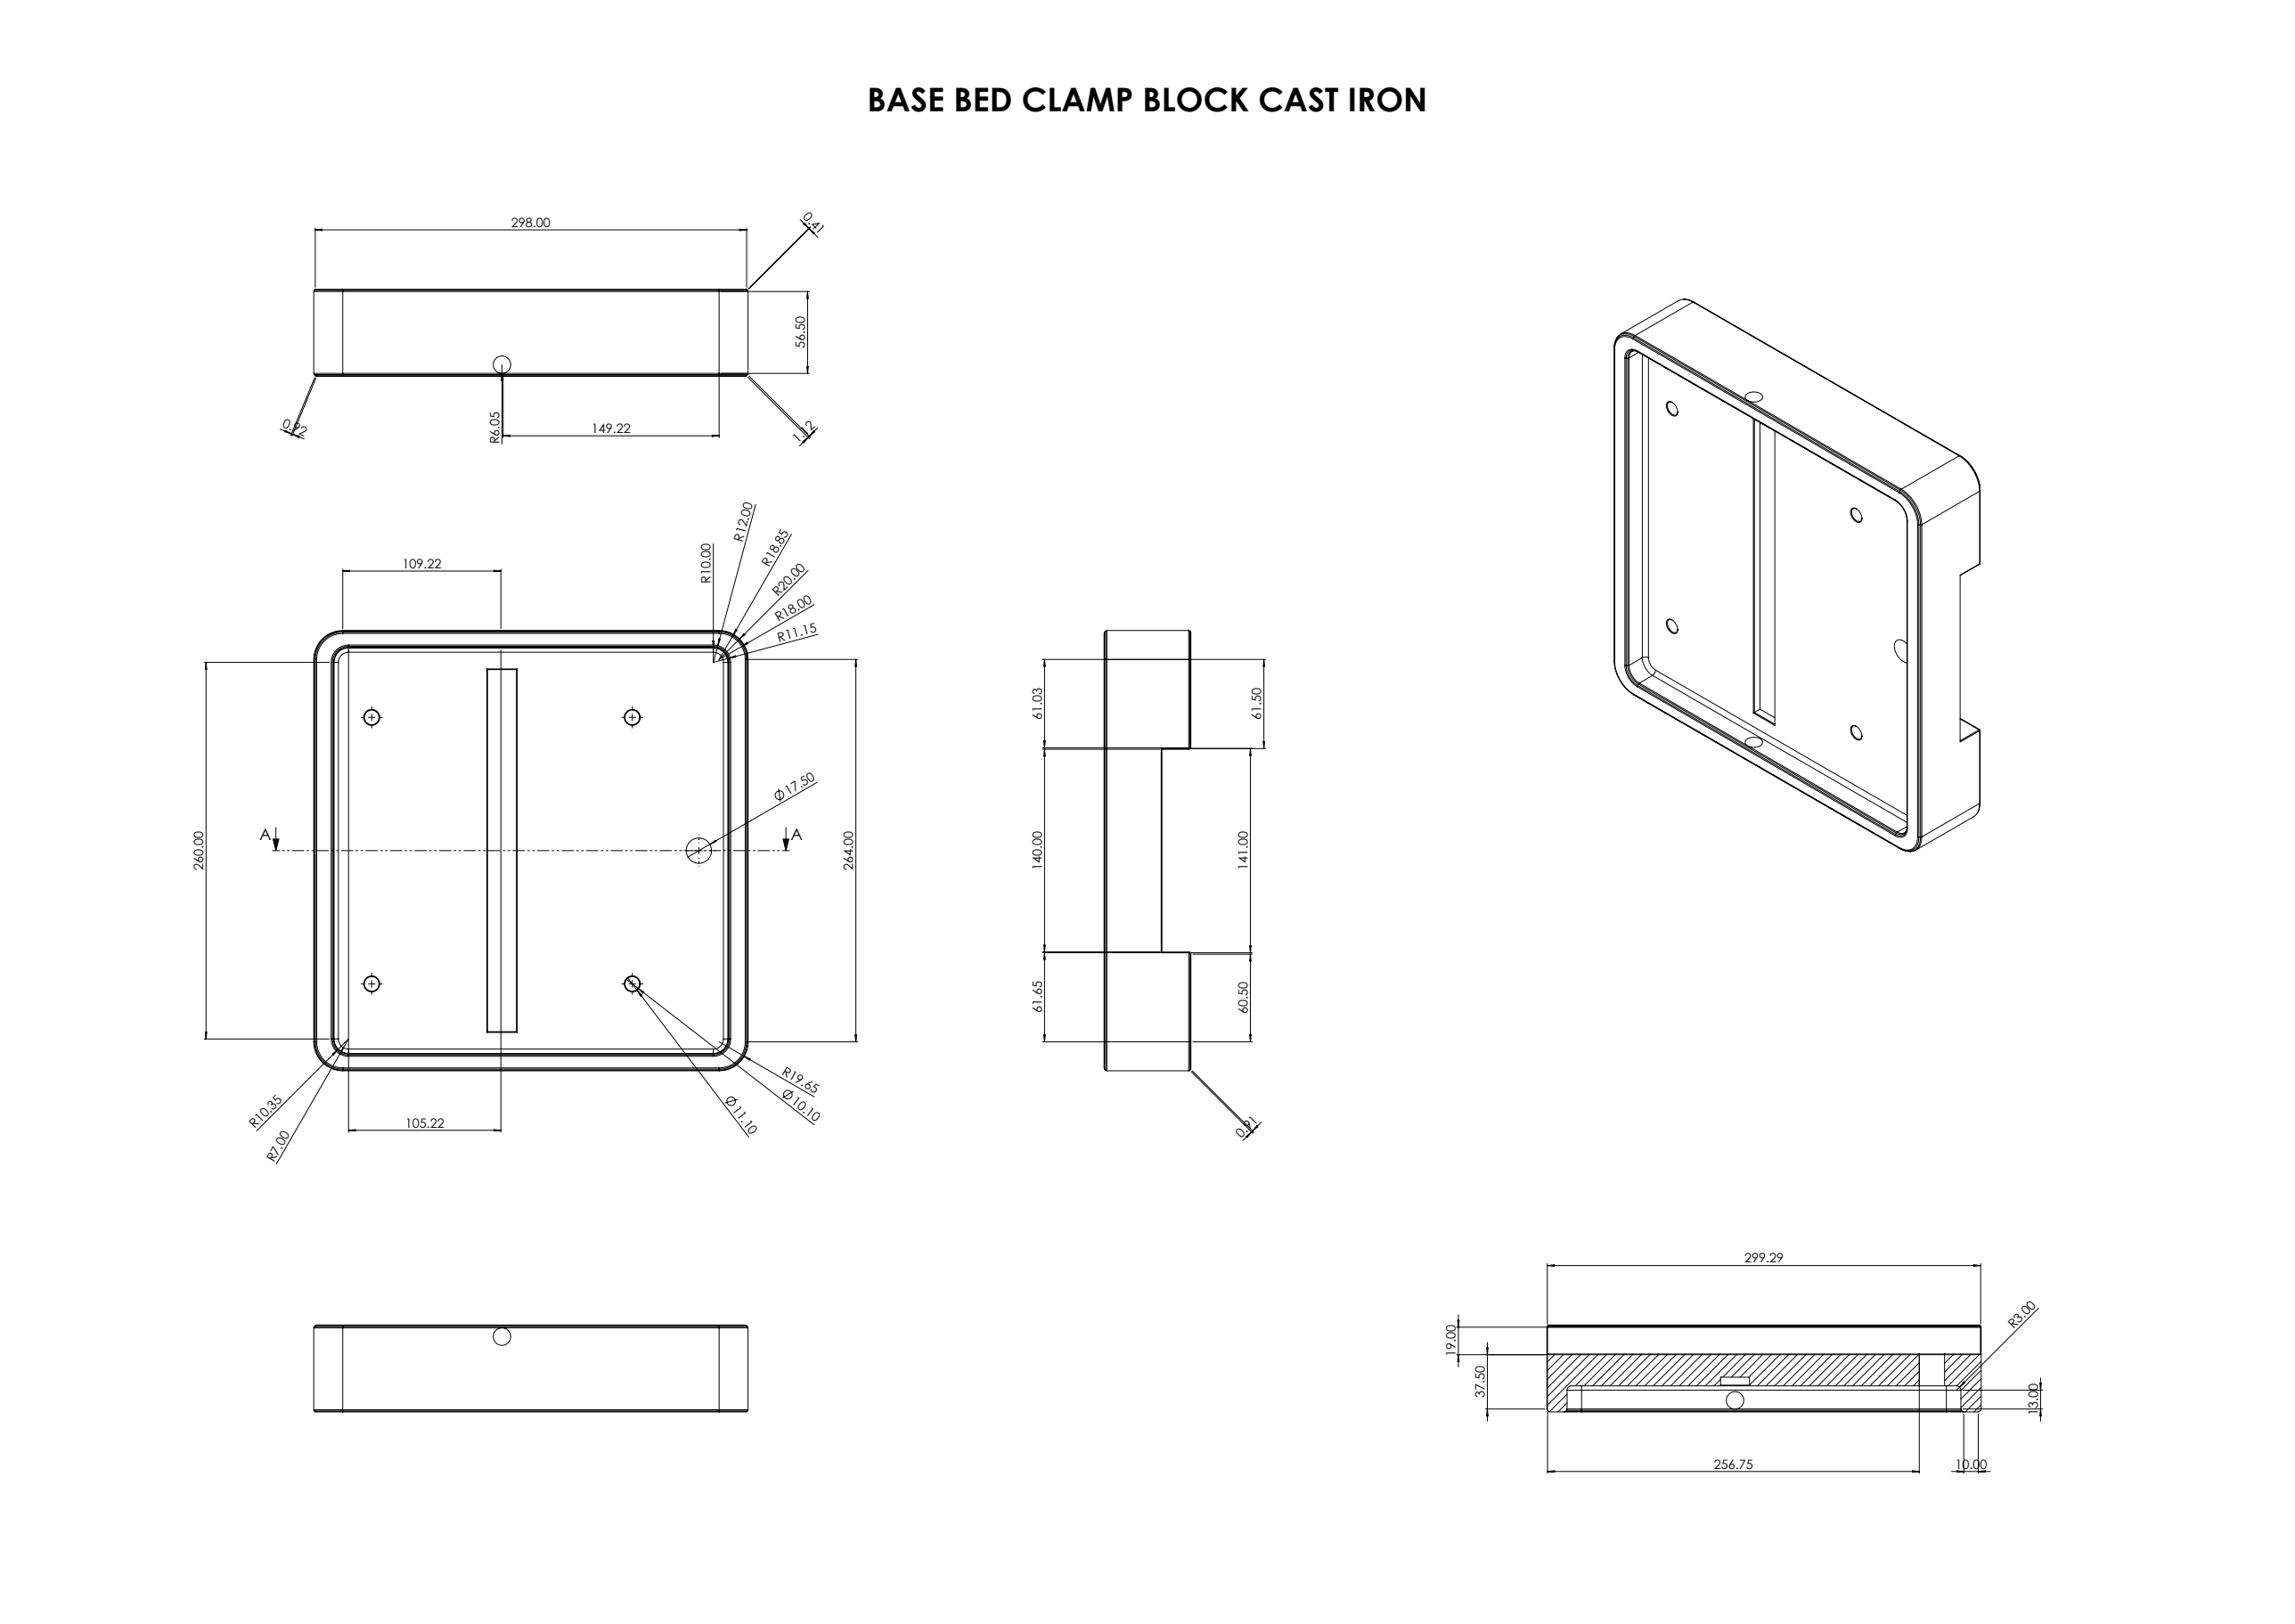
ISO-10303-21;
HEADER;
/* Generated by software containing ST-Developer
 * from STEP Tools, Inc. (www.steptools.com) 
 */

FILE_DESCRIPTION(
/* description */ (''),
/* implementation_level */ '2;1');

FILE_NAME(
/* name */ '01_Base_Bed_Clamp_Block_Cast_Iron.step',
/* time_stamp */ '2026-10-26T03:50:32-07:00',
/* author */ (''),
/* organization */ (''),
/* preprocessor_version */ 'ST-DEVELOPER v20.2',
/* originating_system */ 'Autodesk Translation Framework v15.15.0.0',
/* authorisation */ '');

FILE_SCHEMA (('AUTOMOTIVE_DESIGN { 1 0 10303 214 3 1 1 }'));
ENDSEC;

DATA;
#10=MECHANICAL_DESIGN_GEOMETRIC_PRESENTATION_REPRESENTATION('',(#1039),#76660);
#999=SHAPE_REPRESENTATION_RELATIONSHIP('SRR','None',#76736,#1019);
#1019=ADVANCED_BREP_SHAPE_REPRESENTATION('',(#1059),#76640);
#1039=STYLED_ITEM('',(#76885),#1059);
#1059=MANIFOLD_SOLID_BREP('Base',#26664);
#1079=TOROIDAL_SURFACE('',#27101,0.7,0.3);
#1080=TOROIDAL_SURFACE('',#27107,0.700000000000007,0.3);
#1081=TOROIDAL_SURFACE('',#27111,0.700000000000002,0.3);
#1082=TOROIDAL_SURFACE('',#27115,0.699999999999998,0.3);
#1089=ELLIPSE('',#26967,0.654847281176891,0.605);
#1090=ELLIPSE('',#26976,0.654847281176891,0.605);
#1091=ELLIPSE('',#26995,0.654847281176891,0.605);
#1092=ELLIPSE('',#27030,0.654847281176891,0.605);
#1103=CYLINDRICAL_SURFACE('',#26946,0.505000000000003);
#1104=CYLINDRICAL_SURFACE('',#26950,0.505000000000003);
#1105=CYLINDRICAL_SURFACE('',#26954,0.504999999999999);
#1106=CYLINDRICAL_SURFACE('',#26958,0.504999999999999);
#1107=CYLINDRICAL_SURFACE('',#26985,1.);
#1108=CYLINDRICAL_SURFACE('',#26988,1.00000000000001);
#1109=CYLINDRICAL_SURFACE('',#26993,0.605);
#1110=CYLINDRICAL_SURFACE('',#27043,2.);
#1111=CYLINDRICAL_SURFACE('',#27046,2.);
#1112=CYLINDRICAL_SURFACE('',#27105,0.3);
#1113=CYLINDRICAL_SURFACE('',#27109,0.3);
#1114=CYLINDRICAL_SURFACE('',#27113,0.3);
#1115=CYLINDRICAL_SURFACE('',#27118,0.3);
#1116=CYLINDRICAL_SURFACE('',#27119,0.999999999999998);
#1117=CYLINDRICAL_SURFACE('',#27121,1.);
#1118=CYLINDRICAL_SURFACE('',#27130,2.);
#1119=CYLINDRICAL_SURFACE('',#27131,0.605);
#1120=CYLINDRICAL_SURFACE('',#27132,0.875);
#1121=CYLINDRICAL_SURFACE('',#27140,2.);
#1553=FACE_BOUND('',#4089,.T.);
#1554=FACE_BOUND('',#4092,.T.);
#1555=FACE_BOUND('',#4093,.T.);
#1556=FACE_BOUND('',#4094,.T.);
#1557=FACE_BOUND('',#4095,.T.);
#1558=FACE_BOUND('',#4096,.T.);
#1559=FACE_BOUND('',#4097,.T.);
#1560=FACE_BOUND('',#4194,.T.);
#1656=PLANE('',#26910);
#1657=PLANE('',#26914);
#1658=PLANE('',#26918);
#1659=PLANE('',#26922);
#1660=PLANE('',#26923);
#1661=PLANE('',#26926);
#1662=PLANE('',#26929);
#1663=PLANE('',#26937);
#1664=PLANE('',#26960);
#1665=PLANE('',#26961);
#1666=PLANE('',#26962);
#1667=PLANE('',#26963);
#1668=PLANE('',#26964);
#1669=PLANE('',#26965);
#1670=PLANE('',#26966);
#1671=PLANE('',#26971);
#1672=PLANE('',#26975);
#1673=PLANE('',#26979);
#1674=PLANE('',#26982);
#1675=PLANE('',#26987);
#1676=PLANE('',#26990);
#1677=PLANE('',#26997);
#1678=PLANE('',#26998);
#1679=PLANE('',#26999);
#1680=PLANE('',#27000);
#1681=PLANE('',#27001);
#1682=PLANE('',#27002);
#1683=PLANE('',#27003);
#1684=PLANE('',#27004);
#1685=PLANE('',#27005);
#1686=PLANE('',#27006);
#1687=PLANE('',#27009);
#1688=PLANE('',#27012);
#1689=PLANE('',#27015);
#1690=PLANE('',#27018);
#1691=PLANE('',#27019);
#1692=PLANE('',#27022);
#1693=PLANE('',#27025);
#1694=PLANE('',#27029);
#1695=PLANE('',#27034);
#1696=PLANE('',#27037);
#1697=PLANE('',#27040);
#1698=PLANE('',#27045);
#1699=PLANE('',#27048);
#1700=PLANE('',#27052);
#1701=PLANE('',#27055);
#1702=PLANE('',#27058);
#1703=PLANE('',#27061);
#1704=PLANE('',#27062);
#1705=PLANE('',#27063);
#1706=PLANE('',#27067);
#1707=PLANE('',#27071);
#1708=PLANE('',#27072);
#1709=PLANE('',#27073);
#1710=PLANE('',#27074);
#1711=PLANE('',#27075);
#1712=PLANE('',#27076);
#1713=PLANE('',#27077);
#1714=PLANE('',#27080);
#1715=PLANE('',#27084);
#1716=PLANE('',#27085);
#1717=PLANE('',#27086);
#1718=PLANE('',#27087);
#1719=PLANE('',#27088);
#1720=PLANE('',#27090);
#1721=PLANE('',#27091);
#1722=PLANE('',#27093);
#1723=PLANE('',#27094);
#1724=PLANE('',#27096);
#1725=PLANE('',#27097);
#1726=PLANE('',#27098);
#1727=PLANE('',#27099);
#1728=PLANE('',#27100);
#1729=PLANE('',#27120);
#1730=PLANE('',#27123);
#1731=PLANE('',#27125);
#1732=PLANE('',#27127);
#1733=PLANE('',#27129);
#1734=PLANE('',#27137);
#1735=PLANE('',#27138);
#1736=PLANE('',#27139);
#2524=FACE_OUTER_BOUND('',#4076,.T.);
#2525=FACE_OUTER_BOUND('',#4077,.T.);
#2526=FACE_OUTER_BOUND('',#4078,.T.);
#2527=FACE_OUTER_BOUND('',#4079,.T.);
#2528=FACE_OUTER_BOUND('',#4080,.T.);
#2529=FACE_OUTER_BOUND('',#4081,.T.);
#2530=FACE_OUTER_BOUND('',#4082,.T.);
#2531=FACE_OUTER_BOUND('',#4083,.T.);
#2532=FACE_OUTER_BOUND('',#4084,.T.);
#2533=FACE_OUTER_BOUND('',#4085,.T.);
#2534=FACE_OUTER_BOUND('',#4086,.T.);
#2535=FACE_OUTER_BOUND('',#4087,.T.);
#2536=FACE_OUTER_BOUND('',#4088,.T.);
#2537=FACE_OUTER_BOUND('',#4090,.T.);
#2538=FACE_OUTER_BOUND('',#4091,.T.);
#2539=FACE_OUTER_BOUND('',#4098,.T.);
#2540=FACE_OUTER_BOUND('',#4099,.T.);
#2541=FACE_OUTER_BOUND('',#4100,.T.);
#2542=FACE_OUTER_BOUND('',#4101,.T.);
#2543=FACE_OUTER_BOUND('',#4102,.T.);
#2544=FACE_OUTER_BOUND('',#4103,.T.);
#2545=FACE_OUTER_BOUND('',#4104,.T.);
#2546=FACE_OUTER_BOUND('',#4105,.T.);
#2547=FACE_OUTER_BOUND('',#4106,.T.);
#2548=FACE_OUTER_BOUND('',#4107,.T.);
#2549=FACE_OUTER_BOUND('',#4108,.T.);
#2550=FACE_OUTER_BOUND('',#4109,.T.);
#2551=FACE_OUTER_BOUND('',#4110,.T.);
#2552=FACE_OUTER_BOUND('',#4111,.T.);
#2553=FACE_OUTER_BOUND('',#4112,.T.);
#2554=FACE_OUTER_BOUND('',#4113,.T.);
#2555=FACE_OUTER_BOUND('',#4114,.T.);
#2556=FACE_OUTER_BOUND('',#4115,.T.);
#2557=FACE_OUTER_BOUND('',#4116,.T.);
#2558=FACE_OUTER_BOUND('',#4117,.T.);
#2559=FACE_OUTER_BOUND('',#4118,.T.);
#2560=FACE_OUTER_BOUND('',#4119,.T.);
#2561=FACE_OUTER_BOUND('',#4120,.T.);
#2562=FACE_OUTER_BOUND('',#4121,.T.);
#2563=FACE_OUTER_BOUND('',#4122,.T.);
#2564=FACE_OUTER_BOUND('',#4123,.T.);
#2565=FACE_OUTER_BOUND('',#4124,.T.);
#2566=FACE_OUTER_BOUND('',#4125,.T.);
#2567=FACE_OUTER_BOUND('',#4126,.T.);
#2568=FACE_OUTER_BOUND('',#4127,.T.);
#2569=FACE_OUTER_BOUND('',#4128,.T.);
#2570=FACE_OUTER_BOUND('',#4129,.T.);
#2571=FACE_OUTER_BOUND('',#4130,.T.);
#2572=FACE_OUTER_BOUND('',#4131,.T.);
#2573=FACE_OUTER_BOUND('',#4132,.T.);
#2574=FACE_OUTER_BOUND('',#4133,.T.);
#2575=FACE_OUTER_BOUND('',#4134,.T.);
#2576=FACE_OUTER_BOUND('',#4135,.T.);
#2577=FACE_OUTER_BOUND('',#4136,.T.);
#2578=FACE_OUTER_BOUND('',#4137,.T.);
#2579=FACE_OUTER_BOUND('',#4138,.T.);
#2580=FACE_OUTER_BOUND('',#4139,.T.);
#2581=FACE_OUTER_BOUND('',#4140,.T.);
#2582=FACE_OUTER_BOUND('',#4141,.T.);
#2583=FACE_OUTER_BOUND('',#4142,.T.);
#2584=FACE_OUTER_BOUND('',#4143,.T.);
#2585=FACE_OUTER_BOUND('',#4144,.T.);
#2586=FACE_OUTER_BOUND('',#4145,.T.);
#2587=FACE_OUTER_BOUND('',#4146,.T.);
#2588=FACE_OUTER_BOUND('',#4147,.T.);
#2589=FACE_OUTER_BOUND('',#4148,.T.);
#2590=FACE_OUTER_BOUND('',#4149,.T.);
#2591=FACE_OUTER_BOUND('',#4150,.T.);
#2592=FACE_OUTER_BOUND('',#4151,.T.);
#2593=FACE_OUTER_BOUND('',#4152,.T.);
#2594=FACE_OUTER_BOUND('',#4153,.T.);
#2595=FACE_OUTER_BOUND('',#4154,.T.);
#2596=FACE_OUTER_BOUND('',#4155,.T.);
#2597=FACE_OUTER_BOUND('',#4156,.T.);
#2598=FACE_OUTER_BOUND('',#4157,.T.);
#2599=FACE_OUTER_BOUND('',#4158,.T.);
#2600=FACE_OUTER_BOUND('',#4159,.T.);
#2601=FACE_OUTER_BOUND('',#4160,.T.);
#2602=FACE_OUTER_BOUND('',#4161,.T.);
#2603=FACE_OUTER_BOUND('',#4162,.T.);
#2604=FACE_OUTER_BOUND('',#4163,.T.);
#2605=FACE_OUTER_BOUND('',#4164,.T.);
#2606=FACE_OUTER_BOUND('',#4165,.T.);
#2607=FACE_OUTER_BOUND('',#4166,.T.);
#2608=FACE_OUTER_BOUND('',#4167,.T.);
#2609=FACE_OUTER_BOUND('',#4168,.T.);
#2610=FACE_OUTER_BOUND('',#4169,.T.);
#2611=FACE_OUTER_BOUND('',#4170,.T.);
#2612=FACE_OUTER_BOUND('',#4171,.T.);
#2613=FACE_OUTER_BOUND('',#4172,.T.);
#2614=FACE_OUTER_BOUND('',#4173,.T.);
#2615=FACE_OUTER_BOUND('',#4174,.T.);
#2616=FACE_OUTER_BOUND('',#4175,.T.);
#2617=FACE_OUTER_BOUND('',#4176,.T.);
#2618=FACE_OUTER_BOUND('',#4177,.T.);
#2619=FACE_OUTER_BOUND('',#4178,.T.);
#2620=FACE_OUTER_BOUND('',#4179,.T.);
#2621=FACE_OUTER_BOUND('',#4180,.T.);
#2622=FACE_OUTER_BOUND('',#4181,.T.);
#2623=FACE_OUTER_BOUND('',#4182,.T.);
#2624=FACE_OUTER_BOUND('',#4183,.T.);
#2625=FACE_OUTER_BOUND('',#4184,.T.);
#2626=FACE_OUTER_BOUND('',#4185,.T.);
#2627=FACE_OUTER_BOUND('',#4186,.T.);
#2628=FACE_OUTER_BOUND('',#4187,.T.);
#2629=FACE_OUTER_BOUND('',#4188,.T.);
#2630=FACE_OUTER_BOUND('',#4189,.T.);
#2631=FACE_OUTER_BOUND('',#4190,.T.);
#2632=FACE_OUTER_BOUND('',#4191,.T.);
#2633=FACE_OUTER_BOUND('',#4192,.T.);
#2634=FACE_OUTER_BOUND('',#4193,.T.);
#2635=FACE_OUTER_BOUND('',#4195,.T.);
#2636=FACE_OUTER_BOUND('',#4196,.T.);
#2637=FACE_OUTER_BOUND('',#4197,.T.);
#2638=FACE_OUTER_BOUND('',#4198,.T.);
#2639=FACE_OUTER_BOUND('',#4199,.T.);
#2640=FACE_OUTER_BOUND('',#4200,.T.);
#2641=FACE_OUTER_BOUND('',#4201,.T.);
#2642=FACE_OUTER_BOUND('',#4202,.T.);
#2643=FACE_OUTER_BOUND('',#4203,.T.);
#2644=FACE_OUTER_BOUND('',#4204,.T.);
#2645=FACE_OUTER_BOUND('',#4205,.T.);
#2646=FACE_OUTER_BOUND('',#4206,.T.);
#2647=FACE_OUTER_BOUND('',#4207,.T.);
#2648=FACE_OUTER_BOUND('',#4208,.T.);
#2649=FACE_OUTER_BOUND('',#4209,.T.);
#2650=FACE_OUTER_BOUND('',#4210,.T.);
#2651=FACE_OUTER_BOUND('',#4211,.T.);
#2652=FACE_OUTER_BOUND('',#4212,.T.);
#2653=FACE_OUTER_BOUND('',#4213,.T.);
#2654=FACE_OUTER_BOUND('',#4214,.T.);
#2655=FACE_OUTER_BOUND('',#4215,.T.);
#2656=FACE_OUTER_BOUND('',#4216,.T.);
#2657=FACE_OUTER_BOUND('',#4217,.T.);
#2658=FACE_OUTER_BOUND('',#4218,.T.);
#2659=FACE_OUTER_BOUND('',#4219,.T.);
#2660=FACE_OUTER_BOUND('',#4220,.T.);
#2661=FACE_OUTER_BOUND('',#4221,.T.);
#2662=FACE_OUTER_BOUND('',#4222,.T.);
#2663=FACE_OUTER_BOUND('',#4223,.T.);
#2664=FACE_OUTER_BOUND('',#4224,.T.);
#2665=FACE_OUTER_BOUND('',#4225,.T.);
#2666=FACE_OUTER_BOUND('',#4226,.T.);
#2667=FACE_OUTER_BOUND('',#4227,.T.);
#2668=FACE_OUTER_BOUND('',#4228,.T.);
#2669=FACE_OUTER_BOUND('',#4229,.T.);
#4076=EDGE_LOOP('',(#17185,#17186,#17187,#17188));
#4077=EDGE_LOOP('',(#17189,#17190,#17191,#17192));
#4078=EDGE_LOOP('',(#17193,#17194,#17195,#17196));
#4079=EDGE_LOOP('',(#17197,#17198,#17199,#17200));
#4080=EDGE_LOOP('',(#17201,#17202,#17203,#17204));
#4081=EDGE_LOOP('',(#17205,#17206,#17207,#17208));
#4082=EDGE_LOOP('',(#17209,#17210,#17211,#17212));
#4083=EDGE_LOOP('',(#17213,#17214,#17215,#17216));
#4084=EDGE_LOOP('',(#17217,#17218,#17219,#17220));
#4085=EDGE_LOOP('',(#17221,#17222,#17223,#17224));
#4086=EDGE_LOOP('',(#17225,#17226,#17227,#17228));
#4087=EDGE_LOOP('',(#17229,#17230,#17231,#17232));
#4088=EDGE_LOOP('',(#17233,#17234,#17235,#17236,#17237,#17238,#17239,#17240));
#4089=EDGE_LOOP('',(#17241,#17242,#17243,#17244,#17245,#17246,#17247,#17248));
#4090=EDGE_LOOP('',(#17249,#17250,#17251,#17252));
#4091=EDGE_LOOP('',(#17253,#17254,#17255,#17256,#17257,#17258,#17259,#17260));
#4092=EDGE_LOOP('',(#17261));
#4093=EDGE_LOOP('',(#17262));
#4094=EDGE_LOOP('',(#17263));
#4095=EDGE_LOOP('',(#17264,#17265,#17266,#17267));
#4096=EDGE_LOOP('',(#17268));
#4097=EDGE_LOOP('',(#17269));
#4098=EDGE_LOOP('',(#17270,#17271,#17272,#17273));
#4099=EDGE_LOOP('',(#17274,#17275,#17276,#17277));
#4100=EDGE_LOOP('',(#17278,#17279,#17280,#17281));
#4101=EDGE_LOOP('',(#17282,#17283,#17284,#17285));
#4102=EDGE_LOOP('',(#17286,#17287,#17288,#17289));
#4103=EDGE_LOOP('',(#17290,#17291,#17292,#17293));
#4104=EDGE_LOOP('',(#17294,#17295,#17296,#17297));
#4105=EDGE_LOOP('',(#17298,#17299,#17300,#17301));
#4106=EDGE_LOOP('',(#17302,#17303,#17304,#17305));
#4107=EDGE_LOOP('',(#17306,#17307,#17308,#17309));
#4108=EDGE_LOOP('',(#17310,#17311,#17312,#17313));
#4109=EDGE_LOOP('',(#17314,#17315,#17316,#17317));
#4110=EDGE_LOOP('',(#17318,#17319,#17320,#17321));
#4111=EDGE_LOOP('',(#17322,#17323,#17324,#17325,#17326,#17327));
#4112=EDGE_LOOP('',(#17328,#17329,#17330,#17331));
#4113=EDGE_LOOP('',(#17332,#17333,#17334,#17335));
#4114=EDGE_LOOP('',(#17336,#17337,#17338,#17339));
#4115=EDGE_LOOP('',(#17340,#17341,#17342,#17343,#17344,#17345));
#4116=EDGE_LOOP('',(#17346,#17347,#17348,#17349));
#4117=EDGE_LOOP('',(#17350,#17351,#17352,#17353));
#4118=EDGE_LOOP('',(#17354,#17355,#17356,#17357));
#4119=EDGE_LOOP('',(#17358,#17359,#17360,#17361,#17362,#17363,#17364));
#4120=EDGE_LOOP('',(#17365,#17366,#17367,#17368));
#4121=EDGE_LOOP('',(#17369,#17370,#17371,#17372));
#4122=EDGE_LOOP('',(#17373,#17374,#17375,#17376));
#4123=EDGE_LOOP('',(#17377,#17378,#17379,#17380,#17381,#17382,#17383));
#4124=EDGE_LOOP('',(#17384,#17385,#17386,#17387,#17388,#17389,#17390,#17391));
#4125=EDGE_LOOP('',(#17392,#17393,#17394,#17395,#17396));
#4126=EDGE_LOOP('',(#17397,#17398,#17399,#17400));
#4127=EDGE_LOOP('',(#17401,#17402,#17403,#17404,#17405));
#4128=EDGE_LOOP('',(#17406,#17407,#17408,#17409,#17410,#17411,#17412,#17413));
#4129=EDGE_LOOP('',(#17414,#17415,#17416,#17417,#17418,#17419));
#4130=EDGE_LOOP('',(#17420,#17421,#17422,#17423,#17424));
#4131=EDGE_LOOP('',(#17425,#17426,#17427,#17428,#17429));
#4132=EDGE_LOOP('',(#17430,#17431,#17432,#17433));
#4133=EDGE_LOOP('',(#17434,#17435,#17436,#17437));
#4134=EDGE_LOOP('',(#17438,#17439,#17440,#17441,#17442));
#4135=EDGE_LOOP('',(#17443,#17444,#17445,#17446));
#4136=EDGE_LOOP('',(#17447,#17448,#17449,#17450));
#4137=EDGE_LOOP('',(#17451,#17452,#17453,#17454));
#4138=EDGE_LOOP('',(#17455,#17456,#17457,#17458));
#4139=EDGE_LOOP('',(#17459,#17460,#17461,#17462));
#4140=EDGE_LOOP('',(#17463,#17464,#17465,#17466));
#4141=EDGE_LOOP('',(#17467,#17468,#17469,#17470));
#4142=EDGE_LOOP('',(#17471,#17472,#17473,#17474));
#4143=EDGE_LOOP('',(#17475,#17476,#17477,#17478));
#4144=EDGE_LOOP('',(#17479,#17480,#17481,#17482));
#4145=EDGE_LOOP('',(#17483,#17484,#17485,#17486));
#4146=EDGE_LOOP('',(#17487,#17488,#17489,#17490));
#4147=EDGE_LOOP('',(#17491,#17492,#17493,#17494));
#4148=EDGE_LOOP('',(#17495,#17496,#17497,#17498));
#4149=EDGE_LOOP('',(#17499,#17500,#17501,#17502,#17503,#17504));
#4150=EDGE_LOOP('',(#17505,#17506,#17507,#17508));
#4151=EDGE_LOOP('',(#17509,#17510,#17511,#17512));
#4152=EDGE_LOOP('',(#17513,#17514,#17515,#17516));
#4153=EDGE_LOOP('',(#17517,#17518,#17519,#17520,#17521,#17522));
#4154=EDGE_LOOP('',(#17523,#17524,#17525,#17526));
#4155=EDGE_LOOP('',(#17527,#17528,#17529,#17530,#17531,#17532,#17533));
#4156=EDGE_LOOP('',(#17534,#17535,#17536,#17537));
#4157=EDGE_LOOP('',(#17538,#17539,#17540,#17541,#17542,#17543,#17544,#17545));
#4158=EDGE_LOOP('',(#17546,#17547,#17548,#17549));
#4159=EDGE_LOOP('',(#17550,#17551,#17552,#17553,#17554,#17555,#17556));
#4160=EDGE_LOOP('',(#17557,#17558,#17559,#17560));
#4161=EDGE_LOOP('',(#17561,#17562,#17563,#17564));
#4162=EDGE_LOOP('',(#17565,#17566,#17567,#17568));
#4163=EDGE_LOOP('',(#17569,#17570,#17571,#17572,#17573));
#4164=EDGE_LOOP('',(#17574,#17575,#17576,#17577));
#4165=EDGE_LOOP('',(#17578,#17579,#17580,#17581));
#4166=EDGE_LOOP('',(#17582,#17583,#17584,#17585));
#4167=EDGE_LOOP('',(#17586,#17587,#17588));
#4168=EDGE_LOOP('',(#17589,#17590,#17591));
#4169=EDGE_LOOP('',(#17592,#17593,#17594,#17595));
#4170=EDGE_LOOP('',(#17596,#17597,#17598,#17599));
#4171=EDGE_LOOP('',(#17600,#17601,#17602,#17603));
#4172=EDGE_LOOP('',(#17604,#17605,#17606,#17607));
#4173=EDGE_LOOP('',(#17608,#17609,#17610,#17611));
#4174=EDGE_LOOP('',(#17612,#17613,#17614,#17615));
#4175=EDGE_LOOP('',(#17616,#17617,#17618,#17619));
#4176=EDGE_LOOP('',(#17620,#17621,#17622,#17623));
#4177=EDGE_LOOP('',(#17624,#17625,#17626,#17627));
#4178=EDGE_LOOP('',(#17628,#17629,#17630,#17631));
#4179=EDGE_LOOP('',(#17632,#17633,#17634,#17635));
#4180=EDGE_LOOP('',(#17636,#17637,#17638,#17639));
#4181=EDGE_LOOP('',(#17640,#17641,#17642,#17643));
#4182=EDGE_LOOP('',(#17644,#17645,#17646,#17647));
#4183=EDGE_LOOP('',(#17648,#17649,#17650,#17651));
#4184=EDGE_LOOP('',(#17652,#17653,#17654,#17655));
#4185=EDGE_LOOP('',(#17656,#17657,#17658,#17659));
#4186=EDGE_LOOP('',(#17660,#17661,#17662,#17663));
#4187=EDGE_LOOP('',(#17664,#17665,#17666,#17667));
#4188=EDGE_LOOP('',(#17668,#17669,#17670,#17671));
#4189=EDGE_LOOP('',(#17672,#17673,#17674,#17675));
#4190=EDGE_LOOP('',(#17676,#17677,#17678,#17679));
#4191=EDGE_LOOP('',(#17680,#17681,#17682,#17683));
#4192=EDGE_LOOP('',(#17684,#17685,#17686,#17687));
#4193=EDGE_LOOP('',(#17688,#17689,#17690,#17691));
#4194=EDGE_LOOP('',(#17692));
#4195=EDGE_LOOP('',(#17693,#17694,#17695,#17696));
#4196=EDGE_LOOP('',(#17697,#17698,#17699,#17700,#17701,#17702));
#4197=EDGE_LOOP('',(#17703,#17704,#17705,#17706));
#4198=EDGE_LOOP('',(#17707,#17708,#17709,#17710));
#4199=EDGE_LOOP('',(#17711,#17712,#17713,#17714,#17715,#17716));
#4200=EDGE_LOOP('',(#17717,#17718,#17719,#17720));
#4201=EDGE_LOOP('',(#17721,#17722,#17723,#17724));
#4202=EDGE_LOOP('',(#17725,#17726,#17727,#17728));
#4203=EDGE_LOOP('',(#17729,#17730,#17731,#17732));
#4204=EDGE_LOOP('',(#17733,#17734,#17735,#17736));
#4205=EDGE_LOOP('',(#17737,#17738,#17739,#17740));
#4206=EDGE_LOOP('',(#17741,#17742,#17743,#17744));
#4207=EDGE_LOOP('',(#17745,#17746,#17747,#17748));
#4208=EDGE_LOOP('',(#17749,#17750,#17751,#17752));
#4209=EDGE_LOOP('',(#17753,#17754,#17755,#17756));
#4210=EDGE_LOOP('',(#17757,#17758,#17759,#17760));
#4211=EDGE_LOOP('',(#17761,#17762,#17763,#17764));
#4212=EDGE_LOOP('',(#17765,#17766,#17767,#17768));
#4213=EDGE_LOOP('',(#17769,#17770,#17771,#17772));
#4214=EDGE_LOOP('',(#17773,#17774,#17775,#17776));
#4215=EDGE_LOOP('',(#17777,#17778,#17779,#17780));
#4216=EDGE_LOOP('',(#17781,#17782,#17783,#17784));
#4217=EDGE_LOOP('',(#17785,#17786,#17787,#17788));
#4218=EDGE_LOOP('',(#17789,#17790,#17791,#17792));
#4219=EDGE_LOOP('',(#17793,#17794,#17795,#17796));
#4220=EDGE_LOOP('',(#17797,#17798,#17799,#17800,#17801,#17802,#17803,#17804));
#4221=EDGE_LOOP('',(#17805,#17806,#17807,#17808));
#4222=EDGE_LOOP('',(#17809,#17810,#17811));
#4223=EDGE_LOOP('',(#17812,#17813,#17814));
#4224=EDGE_LOOP('',(#17815,#17816,#17817));
#4225=EDGE_LOOP('',(#17818,#17819,#17820));
#4226=EDGE_LOOP('',(#17821,#17822,#17823,#17824));
#4227=EDGE_LOOP('',(#17825,#17826,#17827,#17828));
#4228=EDGE_LOOP('',(#17829,#17830,#17831,#17832));
#4229=EDGE_LOOP('',(#17833,#17834,#17835,#17836));
#5731=CIRCLE('',#26908,1.11464466094068);
#5732=CIRCLE('',#26909,1.2);
#5733=CIRCLE('',#26912,1.11464466094067);
#5734=CIRCLE('',#26913,1.2);
#5735=CIRCLE('',#26916,1.11464466094067);
#5736=CIRCLE('',#26917,1.2);
#5737=CIRCLE('',#26920,1.11464466094067);
#5738=CIRCLE('',#26921,1.2);
#5739=CIRCLE('',#26925,1.03535533905933);
#5740=CIRCLE('',#26928,1.03535533905933);
#5741=CIRCLE('',#26930,1.8);
#5742=CIRCLE('',#26931,1.8);
#5743=CIRCLE('',#26932,1.8);
#5744=CIRCLE('',#26933,1.80000000000001);
#5745=CIRCLE('',#26935,0.555000000000003);
#5746=CIRCLE('',#26936,0.505000000000003);
#5747=CIRCLE('',#26938,0.7);
#5748=CIRCLE('',#26939,0.699999999999998);
#5749=CIRCLE('',#26940,0.700000000000002);
#5750=CIRCLE('',#26941,0.700000000000007);
#5751=CIRCLE('',#26942,0.555000000000003);
#5752=CIRCLE('',#26943,0.555);
#5753=CIRCLE('',#26944,0.875);
#5754=CIRCLE('',#26945,0.555);
#5755=CIRCLE('',#26947,0.505000000000003);
#5756=CIRCLE('',#26949,0.505000000000003);
#5757=CIRCLE('',#26951,0.505000000000003);
#5758=CIRCLE('',#26953,0.504999999999999);
#5759=CIRCLE('',#26955,0.504999999999999);
#5760=CIRCLE('',#26957,0.504999999999999);
#5761=CIRCLE('',#26959,0.504999999999999);
#5762=CIRCLE('',#26969,1.03535533905933);
#5763=CIRCLE('',#26970,0.999999999999998);
#5764=CIRCLE('',#26973,1.03535533905933);
#5765=CIRCLE('',#26974,1.);
#5766=CIRCLE('',#26978,1.00000000000001);
#5767=CIRCLE('',#26981,1.);
#5768=CIRCLE('',#26983,0.605);
#5769=CIRCLE('',#26984,0.605);
#5770=CIRCLE('',#26986,1.);
#5771=CIRCLE('',#26989,1.00000000000001);
#5772=CIRCLE('',#26991,0.605);
#5773=CIRCLE('',#26992,0.605);
#5774=CIRCLE('',#26994,0.605);
#5775=CIRCLE('',#26996,0.605);
#5776=CIRCLE('',#27008,1.88535533905933);
#5777=CIRCLE('',#27011,1.88535533905933);
#5778=CIRCLE('',#27014,1.88535533905933);
#5779=CIRCLE('',#27017,1.88535533905933);
#5780=CIRCLE('',#27021,1.96464466094067);
#5781=CIRCLE('',#27024,1.96464466094067);
#5782=CIRCLE('',#27027,1.96464466094067);
#5783=CIRCLE('',#27028,2.);
#5784=CIRCLE('',#27032,1.96464466094068);
#5785=CIRCLE('',#27033,2.);
#5786=CIRCLE('',#27036,2.);
#5787=CIRCLE('',#27039,2.);
#5788=CIRCLE('',#27041,0.605);
#5789=CIRCLE('',#27042,0.605);
#5790=CIRCLE('',#27044,2.);
#5791=CIRCLE('',#27047,2.);
#5792=CIRCLE('',#27050,1.96464466094068);
#5793=CIRCLE('',#27051,2.);
#5794=CIRCLE('',#27054,1.96464466094067);
#5795=CIRCLE('',#27057,1.9);
#5796=CIRCLE('',#27060,1.9);
#5797=CIRCLE('',#27065,1.93535533905932);
#5798=CIRCLE('',#27066,1.85);
#5799=CIRCLE('',#27069,1.93535533905933);
#5800=CIRCLE('',#27070,1.85);
#5801=CIRCLE('',#27079,1.96464466094067);
#5802=CIRCLE('',#27082,1.96464466094067);
#5803=CIRCLE('',#27083,2.);
#5804=CIRCLE('',#27095,0.875);
#5805=CIRCLE('',#27102,0.299999999999997);
#5806=CIRCLE('',#27103,0.3);
#5807=CIRCLE('',#27104,1.);
#5808=CIRCLE('',#27106,0.3);
#5809=CIRCLE('',#27108,0.3);
#5810=CIRCLE('',#27110,0.3);
#5811=CIRCLE('',#27112,0.3);
#5812=CIRCLE('',#27114,0.3);
#5813=CIRCLE('',#27116,0.3);
#5814=CIRCLE('',#27117,0.999999999999998);
#6592=LINE('',#36386,#8748);
#6593=LINE('',#36390,#8749);
#6594=LINE('',#36395,#8750);
#6595=LINE('',#36396,#8751);
#6596=LINE('',#36397,#8752);
#6597=LINE('',#36401,#8753);
#6598=LINE('',#36407,#8754);
#6599=LINE('',#36408,#8755);
#6600=LINE('',#36409,#8756);
#6601=LINE('',#36413,#8757);
#6602=LINE('',#36419,#8758);
#6603=LINE('',#36420,#8759);
#6604=LINE('',#36421,#8760);
#6605=LINE('',#36425,#8761);
#6606=LINE('',#36429,#8762);
#6607=LINE('',#36430,#8763);
#6608=LINE('',#36433,#8764);
#6609=LINE('',#36435,#8765);
#6610=LINE('',#36436,#8766);
#6611=LINE('',#36439,#8767);
#6612=LINE('',#36443,#8768);
#6613=LINE('',#36444,#8769);
#6614=LINE('',#36447,#8770);
#6615=LINE('',#36454,#8771);
#6616=LINE('',#36458,#8772);
#6617=LINE('',#36462,#8773);
#6618=LINE('',#36465,#8774);
#6619=LINE('',#36470,#8775);
#6620=LINE('',#36477,#8776);
#6621=LINE('',#36481,#8777);
#6622=LINE('',#36485,#8778);
#6623=LINE('',#36488,#8779);
#6624=LINE('',#36497,#8780);
#6625=LINE('',#36499,#8781);
#6626=LINE('',#36501,#8782);
#6627=LINE('',#36502,#8783);
#6628=LINE('',#36508,#8784);
#6629=LINE('',#36511,#8785);
#6630=LINE('',#36516,#8786);
#6631=LINE('',#36519,#8787);
#6632=LINE('',#36524,#8788);
#6633=LINE('',#36527,#8789);
#6634=LINE('',#36532,#8790);
#6635=LINE('',#36535,#8791);
#6636=LINE('',#36537,#8792);
#6637=LINE('',#36538,#8793);
#6638=LINE('',#36541,#8794);
#6639=LINE('',#36543,#8795);
#6640=LINE('',#36544,#8796);
#6641=LINE('',#36546,#8797);
#6642=LINE('',#36548,#8798);
#6643=LINE('',#36551,#8799);
#6644=LINE('',#36553,#8800);
#6645=LINE('',#36554,#8801);
#6646=LINE('',#36557,#8802);
#6647=LINE('',#36558,#8803);
#6648=LINE('',#36564,#8804);
#6649=LINE('',#36565,#8805);
#6650=LINE('',#36567,#8806);
#6651=LINE('',#36568,#8807);
#6652=LINE('',#36572,#8808);
#6653=LINE('',#36578,#8809);
#6654=LINE('',#36579,#8810);
#6655=LINE('',#36580,#8811);
#6656=LINE('',#36584,#8812);
#6657=LINE('',#36592,#8813);
#6658=LINE('',#36593,#8814);
#6659=LINE('',#36594,#8815);
#6660=LINE('',#36595,#8816);
#6661=LINE('',#36598,#8817);
#6662=LINE('',#36602,#8818);
#6663=LINE('',#36603,#8819);
#6664=LINE('',#36608,#8820);
#6665=LINE('',#36610,#8821);
#6666=LINE('',#36611,#8822);
#6667=LINE('',#36617,#8823);
#6668=LINE('',#36621,#8824);
#6669=LINE('',#36622,#8825);
#6670=LINE('',#36625,#8826);
#6671=LINE('',#36632,#8827);
#6672=LINE('',#36633,#8828);
#6673=LINE('',#36636,#8829);
#6674=LINE('',#36645,#8830);
#6675=LINE('',#36647,#8831);
#6676=LINE('',#36649,#8832);
#6677=LINE('',#36651,#8833);
#6678=LINE('',#36652,#8834);
#6679=LINE('',#36655,#8835);
#6680=LINE('',#36657,#8836);
#6681=LINE('',#36658,#8837);
#6682=LINE('',#36661,#8838);
#6683=LINE('',#36663,#8839);
#6684=LINE('',#36665,#8840);
#6685=LINE('',#36666,#8841);
#6686=LINE('',#36669,#8842);
#6687=LINE('',#36671,#8843);
#6688=LINE('',#36673,#8844);
#6689=LINE('',#36675,#8845);
#6690=LINE('',#36676,#8846);
#6691=LINE('',#36679,#8847);
#6692=LINE('',#36681,#8848);
#6693=LINE('',#36683,#8849);
#6694=LINE('',#36684,#8850);
#6695=LINE('',#36687,#8851);
#6696=LINE('',#36689,#8852);
#6697=LINE('',#36691,#8853);
#6698=LINE('',#36692,#8854);
#6699=LINE('',#36695,#8855);
#6700=LINE('',#36697,#8856);
#6701=LINE('',#36698,#8857);
#6702=LINE('',#36701,#8858);
#6703=LINE('',#36703,#8859);
#6704=LINE('',#36704,#8860);
#6705=LINE('',#36707,#8861);
#6706=LINE('',#36709,#8862);
#6707=LINE('',#36710,#8863);
#6708=LINE('',#36713,#8864);
#6709=LINE('',#36714,#8865);
#6710=LINE('',#36717,#8866);
#6711=LINE('',#36720,#8867);
#6712=LINE('',#36723,#8868);
#6713=LINE('',#36724,#8869);
#6714=LINE('',#36727,#8870);
#6715=LINE('',#36731,#8871);
#6716=LINE('',#36732,#8872);
#6717=LINE('',#36735,#8873);
#6718=LINE('',#36739,#8874);
#6719=LINE('',#36740,#8875);
#6720=LINE('',#36743,#8876);
#6721=LINE('',#36746,#8877);
#6722=LINE('',#36749,#8878);
#6723=LINE('',#36751,#8879);
#6724=LINE('',#36752,#8880);
#6725=LINE('',#36755,#8881);
#6726=LINE('',#36759,#8882);
#6727=LINE('',#36760,#8883);
#6728=LINE('',#36763,#8884);
#6729=LINE('',#36767,#8885);
#6730=LINE('',#36769,#8886);
#6731=LINE('',#36770,#8887);
#6732=LINE('',#36774,#8888);
#6733=LINE('',#36782,#8889);
#6734=LINE('',#36784,#8890);
#6735=LINE('',#36785,#8891);
#6736=LINE('',#36786,#8892);
#6737=LINE('',#36789,#8893);
#6738=LINE('',#36793,#8894);
#6739=LINE('',#36794,#8895);
#6740=LINE('',#36797,#8896);
#6741=LINE('',#36801,#8897);
#6742=LINE('',#36802,#8898);
#6743=LINE('',#36803,#8899);
#6744=LINE('',#36808,#8900);
#6745=LINE('',#36810,#8901);
#6746=LINE('',#36811,#8902);
#6747=LINE('',#36816,#8903);
#6748=LINE('',#36820,#8904);
#6749=LINE('',#36822,#8905);
#6750=LINE('',#36824,#8906);
#6751=LINE('',#36825,#8907);
#6752=LINE('',#36828,#8908);
#6753=LINE('',#36832,#8909);
#6754=LINE('',#36833,#8910);
#6755=LINE('',#36836,#8911);
#6756=LINE('',#36841,#8912);
#6757=LINE('',#36842,#8913);
#6758=LINE('',#36847,#8914);
#6759=LINE('',#36848,#8915);
#6760=LINE('',#36851,#8916);
#6761=LINE('',#36855,#8917);
#6762=LINE('',#36856,#8918);
#6763=LINE('',#36862,#8919);
#6764=LINE('',#36864,#8920);
#6765=LINE('',#36865,#8921);
#6766=LINE('',#36869,#8922);
#6767=LINE('',#36871,#8923);
#6768=LINE('',#36872,#8924);
#6769=LINE('',#36876,#8925);
#6770=LINE('',#36877,#8926);
#6771=LINE('',#36878,#8927);
#6772=LINE('',#36882,#8928);
#6773=LINE('',#36888,#8929);
#6774=LINE('',#36889,#8930);
#6775=LINE('',#36890,#8931);
#6776=LINE('',#36894,#8932);
#6777=LINE('',#36898,#8933);
#6778=LINE('',#36899,#8934);
#6779=LINE('',#36901,#8935);
#6780=LINE('',#36902,#8936);
#6781=LINE('',#36906,#8937);
#6782=LINE('',#36907,#8938);
#6783=LINE('',#36909,#8939);
#6784=LINE('',#36910,#8940);
#6785=LINE('',#36914,#8941);
#6786=LINE('',#36915,#8942);
#6787=LINE('',#36917,#8943);
#6788=LINE('',#36918,#8944);
#6789=LINE('',#36921,#8945);
#6790=LINE('',#36922,#8946);
#6791=LINE('',#36924,#8947);
#6792=LINE('',#36927,#8948);
#6793=LINE('',#36928,#8949);
#6794=LINE('',#36931,#8950);
#6795=LINE('',#36935,#8951);
#6796=LINE('',#36936,#8952);
#6797=LINE('',#36939,#8953);
#6798=LINE('',#36943,#8954);
#6799=LINE('',#36945,#8955);
#6800=LINE('',#36946,#8956);
#6801=LINE('',#36948,#8957);
#6802=LINE('',#36949,#8958);
#6803=LINE('',#36951,#8959);
#6804=LINE('',#36953,#8960);
#6805=LINE('',#36954,#8961);
#6806=LINE('',#36956,#8962);
#6807=LINE('',#36957,#8963);
#6808=LINE('',#36959,#8964);
#6809=LINE('',#36961,#8965);
#6810=LINE('',#36964,#8966);
#6811=LINE('',#36966,#8967);
#6812=LINE('',#36994,#8968);
#6813=LINE('',#36996,#8969);
#6814=LINE('',#36998,#8970);
#6815=LINE('',#37001,#8971);
#6816=LINE('',#37003,#8972);
#6817=LINE('',#37005,#8973);
#6818=LINE('',#37008,#8974);
#6819=LINE('',#37010,#8975);
#6820=LINE('',#37012,#8976);
#6821=LINE('',#37016,#8977);
#6822=LINE('',#37018,#8978);
#6823=LINE('',#37021,#8979);
#6824=LINE('',#37024,#8980);
#6825=LINE('',#37027,#8981);
#6826=LINE('',#37030,#8982);
#6827=LINE('',#37033,#8983);
#6828=LINE('',#37034,#8984);
#6829=LINE('',#37036,#8985);
#8748=VECTOR('',#29351,1.);
#8749=VECTOR('',#29354,1.);
#8750=VECTOR('',#29359,1.);
#8751=VECTOR('',#29360,1.);
#8752=VECTOR('',#29361,1.);
#8753=VECTOR('',#29364,1.);
#8754=VECTOR('',#29371,1.);
#8755=VECTOR('',#29372,1.);
#8756=VECTOR('',#29373,1.);
#8757=VECTOR('',#29376,1.);
#8758=VECTOR('',#29383,1.);
#8759=VECTOR('',#29384,1.);
#8760=VECTOR('',#29385,1.);
#8761=VECTOR('',#29388,1.);
#8762=VECTOR('',#29395,1.);
#8763=VECTOR('',#29396,1.);
#8764=VECTOR('',#29399,1.);
#8765=VECTOR('',#29400,1.);
#8766=VECTOR('',#29401,1.);
#8767=VECTOR('',#29404,1.);
#8768=VECTOR('',#29409,1.);
#8769=VECTOR('',#29410,1.);
#8770=VECTOR('',#29413,1.);
#8771=VECTOR('',#29420,1.);
#8772=VECTOR('',#29423,1.);
#8773=VECTOR('',#29426,1.);
#8774=VECTOR('',#29429,1.);
#8775=VECTOR('',#29434,0.530000000000003);
#8776=VECTOR('',#29441,1.);
#8777=VECTOR('',#29444,1.);
#8778=VECTOR('',#29447,1.);
#8779=VECTOR('',#29450,1.);
#8780=VECTOR('',#29457,1.);
#8781=VECTOR('',#29458,1.);
#8782=VECTOR('',#29459,1.);
#8783=VECTOR('',#29460,1.);
#8784=VECTOR('',#29467,0.505000000000003);
#8785=VECTOR('',#29470,0.530000000000003);
#8786=VECTOR('',#29477,0.505000000000003);
#8787=VECTOR('',#29480,0.529999999999999);
#8788=VECTOR('',#29487,0.504999999999999);
#8789=VECTOR('',#29490,0.529999999999999);
#8790=VECTOR('',#29497,0.504999999999999);
#8791=VECTOR('',#29500,1.);
#8792=VECTOR('',#29501,1.);
#8793=VECTOR('',#29502,1.);
#8794=VECTOR('',#29505,1.);
#8795=VECTOR('',#29506,1.);
#8796=VECTOR('',#29507,1.);
#8797=VECTOR('',#29510,1.);
#8798=VECTOR('',#29513,1.);
#8799=VECTOR('',#29516,1.);
#8800=VECTOR('',#29517,1.);
#8801=VECTOR('',#29518,1.);
#8802=VECTOR('',#29521,1.);
#8803=VECTOR('',#29522,1.);
#8804=VECTOR('',#29527,1.);
#8805=VECTOR('',#29528,1.);
#8806=VECTOR('',#29529,1.);
#8807=VECTOR('',#29530,1.);
#8808=VECTOR('',#29533,1.);
#8809=VECTOR('',#29540,1.);
#8810=VECTOR('',#29541,1.);
#8811=VECTOR('',#29542,1.);
#8812=VECTOR('',#29545,1.);
#8813=VECTOR('',#29554,1.);
#8814=VECTOR('',#29555,1.);
#8815=VECTOR('',#29556,1.);
#8816=VECTOR('',#29557,1.);
#8817=VECTOR('',#29560,1.);
#8818=VECTOR('',#29565,1.);
#8819=VECTOR('',#29566,1.);
#8820=VECTOR('',#29573,1.);
#8821=VECTOR('',#29574,1.);
#8822=VECTOR('',#29575,1.);
#8823=VECTOR('',#29582,1.);
#8824=VECTOR('',#29587,1.);
#8825=VECTOR('',#29588,1.);
#8826=VECTOR('',#29591,1.);
#8827=VECTOR('',#29600,1.);
#8828=VECTOR('',#29601,1.);
#8829=VECTOR('',#29604,0.605);
#8830=VECTOR('',#29613,1.);
#8831=VECTOR('',#29614,1.);
#8832=VECTOR('',#29615,1.);
#8833=VECTOR('',#29616,1.);
#8834=VECTOR('',#29617,1.);
#8835=VECTOR('',#29620,1.);
#8836=VECTOR('',#29621,1.);
#8837=VECTOR('',#29622,1.);
#8838=VECTOR('',#29625,1.);
#8839=VECTOR('',#29626,1.);
#8840=VECTOR('',#29627,1.);
#8841=VECTOR('',#29628,1.);
#8842=VECTOR('',#29631,1.);
#8843=VECTOR('',#29632,1.);
#8844=VECTOR('',#29633,1.);
#8845=VECTOR('',#29634,1.);
#8846=VECTOR('',#29635,1.);
#8847=VECTOR('',#29638,1.);
#8848=VECTOR('',#29639,1.);
#8849=VECTOR('',#29640,1.);
#8850=VECTOR('',#29641,1.);
#8851=VECTOR('',#29644,1.);
#8852=VECTOR('',#29645,1.);
#8853=VECTOR('',#29646,1.);
#8854=VECTOR('',#29647,1.);
#8855=VECTOR('',#29650,1.);
#8856=VECTOR('',#29651,1.);
#8857=VECTOR('',#29652,1.);
#8858=VECTOR('',#29655,1.);
#8859=VECTOR('',#29656,1.);
#8860=VECTOR('',#29657,1.);
#8861=VECTOR('',#29660,1.);
#8862=VECTOR('',#29661,1.);
#8863=VECTOR('',#29662,1.);
#8864=VECTOR('',#29665,1.);
#8865=VECTOR('',#29666,1.);
#8866=VECTOR('',#29669,1.);
#8867=VECTOR('',#29672,1.);
#8868=VECTOR('',#29675,1.);
#8869=VECTOR('',#29676,1.);
#8870=VECTOR('',#29679,1.);
#8871=VECTOR('',#29684,1.);
#8872=VECTOR('',#29685,1.);
#8873=VECTOR('',#29688,1.);
#8874=VECTOR('',#29693,1.);
#8875=VECTOR('',#29694,1.);
#8876=VECTOR('',#29697,1.);
#8877=VECTOR('',#29702,1.);
#8878=VECTOR('',#29705,1.);
#8879=VECTOR('',#29706,1.);
#8880=VECTOR('',#29707,1.);
#8881=VECTOR('',#29710,1.);
#8882=VECTOR('',#29715,1.);
#8883=VECTOR('',#29716,1.);
#8884=VECTOR('',#29719,1.);
#8885=VECTOR('',#29724,1.);
#8886=VECTOR('',#29725,1.);
#8887=VECTOR('',#29726,1.);
#8888=VECTOR('',#29729,1.);
#8889=VECTOR('',#29738,1.);
#8890=VECTOR('',#29739,1.);
#8891=VECTOR('',#29740,1.);
#8892=VECTOR('',#29741,1.);
#8893=VECTOR('',#29744,1.);
#8894=VECTOR('',#29751,1.);
#8895=VECTOR('',#29752,1.);
#8896=VECTOR('',#29755,1.);
#8897=VECTOR('',#29760,1.);
#8898=VECTOR('',#29761,1.);
#8899=VECTOR('',#29762,1.);
#8900=VECTOR('',#29769,1.);
#8901=VECTOR('',#29770,1.);
#8902=VECTOR('',#29771,1.);
#8903=VECTOR('',#29778,1.);
#8904=VECTOR('',#29783,1.);
#8905=VECTOR('',#29784,1.);
#8906=VECTOR('',#29785,1.);
#8907=VECTOR('',#29786,1.);
#8908=VECTOR('',#29789,1.);
#8909=VECTOR('',#29794,1.);
#8910=VECTOR('',#29795,1.);
#8911=VECTOR('',#29798,1.);
#8912=VECTOR('',#29805,1.);
#8913=VECTOR('',#29806,1.);
#8914=VECTOR('',#29813,1.);
#8915=VECTOR('',#29814,1.);
#8916=VECTOR('',#29817,1.);
#8917=VECTOR('',#29822,1.);
#8918=VECTOR('',#29823,1.);
#8919=VECTOR('',#29830,1.);
#8920=VECTOR('',#29831,1.);
#8921=VECTOR('',#29832,1.);
#8922=VECTOR('',#29835,1.);
#8923=VECTOR('',#29836,1.);
#8924=VECTOR('',#29837,1.);
#8925=VECTOR('',#29840,1.);
#8926=VECTOR('',#29841,1.);
#8927=VECTOR('',#29842,1.);
#8928=VECTOR('',#29845,1.);
#8929=VECTOR('',#29852,1.);
#8930=VECTOR('',#29853,1.);
#8931=VECTOR('',#29854,1.);
#8932=VECTOR('',#29857,1.);
#8933=VECTOR('',#29864,1.);
#8934=VECTOR('',#29865,1.);
#8935=VECTOR('',#29868,1.);
#8936=VECTOR('',#29869,1.);
#8937=VECTOR('',#29872,1.);
#8938=VECTOR('',#29873,1.);
#8939=VECTOR('',#29874,1.);
#8940=VECTOR('',#29875,1.);
#8941=VECTOR('',#29878,1.);
#8942=VECTOR('',#29879,1.);
#8943=VECTOR('',#29880,1.);
#8944=VECTOR('',#29881,1.);
#8945=VECTOR('',#29884,1.);
#8946=VECTOR('',#29885,1.);
#8947=VECTOR('',#29888,1.);
#8948=VECTOR('',#29891,1.);
#8949=VECTOR('',#29892,1.);
#8950=VECTOR('',#29895,1.);
#8951=VECTOR('',#29900,1.);
#8952=VECTOR('',#29901,1.);
#8953=VECTOR('',#29904,1.);
#8954=VECTOR('',#29911,1.);
#8955=VECTOR('',#29914,1.);
#8956=VECTOR('',#29915,1.);
#8957=VECTOR('',#29918,1.);
#8958=VECTOR('',#29919,1.);
#8959=VECTOR('',#29922,1.);
#8960=VECTOR('',#29925,1.);
#8961=VECTOR('',#29926,1.);
#8962=VECTOR('',#29929,1.);
#8963=VECTOR('',#29930,1.);
#8964=VECTOR('',#29933,1.);
#8965=VECTOR('',#29936,1.);
#8966=VECTOR('',#29941,1.);
#8967=VECTOR('',#29944,1.);
#8968=VECTOR('',#29993,1.);
#8969=VECTOR('',#29996,1.);
#8970=VECTOR('',#29999,1.);
#8971=VECTOR('',#30004,1.);
#8972=VECTOR('',#30007,1.);
#8973=VECTOR('',#30010,1.);
#8974=VECTOR('',#30015,1.);
#8975=VECTOR('',#30018,1.);
#8976=VECTOR('',#30021,1.);
#8977=VECTOR('',#30028,0.605);
#8978=VECTOR('',#30031,0.875);
#8979=VECTOR('',#30034,0.252500000000001);
#8980=VECTOR('',#30037,0.252500000000001);
#8981=VECTOR('',#30040,0.2525);
#8982=VECTOR('',#30043,0.2525);
#8983=VECTOR('',#30046,1.);
#8984=VECTOR('',#30047,1.);
#8985=VECTOR('',#30050,1.);
#10904=VERTEX_POINT('',#36384);
#10905=VERTEX_POINT('',#36385);
#10906=VERTEX_POINT('',#36387);
#10907=VERTEX_POINT('',#36389);
#10908=VERTEX_POINT('',#36393);
#10909=VERTEX_POINT('',#36394);
#10910=VERTEX_POINT('',#36399);
#10911=VERTEX_POINT('',#36400);
#10912=VERTEX_POINT('',#36405);
#10913=VERTEX_POINT('',#36406);
#10914=VERTEX_POINT('',#36411);
#10915=VERTEX_POINT('',#36412);
#10916=VERTEX_POINT('',#36417);
#10917=VERTEX_POINT('',#36418);
#10918=VERTEX_POINT('',#36423);
#10919=VERTEX_POINT('',#36424);
#10920=VERTEX_POINT('',#36432);
#10921=VERTEX_POINT('',#36434);
#10922=VERTEX_POINT('',#36438);
#10923=VERTEX_POINT('',#36442);
#10924=VERTEX_POINT('',#36446);
#10925=VERTEX_POINT('',#36450);
#10926=VERTEX_POINT('',#36451);
#10927=VERTEX_POINT('',#36453);
#10928=VERTEX_POINT('',#36455);
#10929=VERTEX_POINT('',#36457);
#10930=VERTEX_POINT('',#36459);
#10931=VERTEX_POINT('',#36461);
#10932=VERTEX_POINT('',#36463);
#10933=VERTEX_POINT('',#36467);
#10934=VERTEX_POINT('',#36469);
#10935=VERTEX_POINT('',#36473);
#10936=VERTEX_POINT('',#36474);
#10937=VERTEX_POINT('',#36476);
#10938=VERTEX_POINT('',#36478);
#10939=VERTEX_POINT('',#36480);
#10940=VERTEX_POINT('',#36482);
#10941=VERTEX_POINT('',#36484);
#10942=VERTEX_POINT('',#36486);
#10943=VERTEX_POINT('',#36489);
#10944=VERTEX_POINT('',#36491);
#10945=VERTEX_POINT('',#36493);
#10946=VERTEX_POINT('',#36495);
#10947=VERTEX_POINT('',#36496);
#10948=VERTEX_POINT('',#36498);
#10949=VERTEX_POINT('',#36500);
#10950=VERTEX_POINT('',#36503);
#10951=VERTEX_POINT('',#36506);
#10952=VERTEX_POINT('',#36510);
#10953=VERTEX_POINT('',#36514);
#10954=VERTEX_POINT('',#36518);
#10955=VERTEX_POINT('',#36522);
#10956=VERTEX_POINT('',#36526);
#10957=VERTEX_POINT('',#36530);
#10958=VERTEX_POINT('',#36534);
#10959=VERTEX_POINT('',#36536);
#10960=VERTEX_POINT('',#36540);
#10961=VERTEX_POINT('',#36542);
#10962=VERTEX_POINT('',#36550);
#10963=VERTEX_POINT('',#36552);
#10964=VERTEX_POINT('',#36556);
#10965=VERTEX_POINT('',#36560);
#10966=VERTEX_POINT('',#36561);
#10967=VERTEX_POINT('',#36563);
#10968=VERTEX_POINT('',#36566);
#10969=VERTEX_POINT('',#36570);
#10970=VERTEX_POINT('',#36571);
#10971=VERTEX_POINT('',#36576);
#10972=VERTEX_POINT('',#36577);
#10973=VERTEX_POINT('',#36582);
#10974=VERTEX_POINT('',#36583);
#10975=VERTEX_POINT('',#36588);
#10976=VERTEX_POINT('',#36589);
#10977=VERTEX_POINT('',#36591);
#10978=VERTEX_POINT('',#36597);
#10979=VERTEX_POINT('',#36601);
#10980=VERTEX_POINT('',#36607);
#10981=VERTEX_POINT('',#36609);
#10982=VERTEX_POINT('',#36612);
#10983=VERTEX_POINT('',#36616);
#10984=VERTEX_POINT('',#36620);
#10985=VERTEX_POINT('',#36624);
#10986=VERTEX_POINT('',#36628);
#10987=VERTEX_POINT('',#36631);
#10988=VERTEX_POINT('',#36635);
#10989=VERTEX_POINT('',#36637);
#10990=VERTEX_POINT('',#36639);
#10991=VERTEX_POINT('',#36643);
#10992=VERTEX_POINT('',#36644);
#10993=VERTEX_POINT('',#36646);
#10994=VERTEX_POINT('',#36648);
#10995=VERTEX_POINT('',#36650);
#10996=VERTEX_POINT('',#36654);
#10997=VERTEX_POINT('',#36656);
#10998=VERTEX_POINT('',#36660);
#10999=VERTEX_POINT('',#36662);
#11000=VERTEX_POINT('',#36664);
#11001=VERTEX_POINT('',#36668);
#11002=VERTEX_POINT('',#36670);
#11003=VERTEX_POINT('',#36672);
#11004=VERTEX_POINT('',#36674);
#11005=VERTEX_POINT('',#36678);
#11006=VERTEX_POINT('',#36680);
#11007=VERTEX_POINT('',#36682);
#11008=VERTEX_POINT('',#36686);
#11009=VERTEX_POINT('',#36688);
#11010=VERTEX_POINT('',#36690);
#11011=VERTEX_POINT('',#36694);
#11012=VERTEX_POINT('',#36696);
#11013=VERTEX_POINT('',#36700);
#11014=VERTEX_POINT('',#36702);
#11015=VERTEX_POINT('',#36706);
#11016=VERTEX_POINT('',#36708);
#11017=VERTEX_POINT('',#36712);
#11018=VERTEX_POINT('',#36716);
#11019=VERTEX_POINT('',#36718);
#11020=VERTEX_POINT('',#36722);
#11021=VERTEX_POINT('',#36726);
#11022=VERTEX_POINT('',#36730);
#11023=VERTEX_POINT('',#36734);
#11024=VERTEX_POINT('',#36738);
#11025=VERTEX_POINT('',#36742);
#11026=VERTEX_POINT('',#36748);
#11027=VERTEX_POINT('',#36750);
#11028=VERTEX_POINT('',#36754);
#11029=VERTEX_POINT('',#36758);
#11030=VERTEX_POINT('',#36762);
#11031=VERTEX_POINT('',#36766);
#11032=VERTEX_POINT('',#36768);
#11033=VERTEX_POINT('',#36772);
#11034=VERTEX_POINT('',#36773);
#11035=VERTEX_POINT('',#36778);
#11036=VERTEX_POINT('',#36779);
#11037=VERTEX_POINT('',#36781);
#11038=VERTEX_POINT('',#36783);
#11039=VERTEX_POINT('',#36788);
#11040=VERTEX_POINT('',#36796);
#11041=VERTEX_POINT('',#36800);
#11042=VERTEX_POINT('',#36807);
#11043=VERTEX_POINT('',#36809);
#11044=VERTEX_POINT('',#36812);
#11045=VERTEX_POINT('',#36819);
#11046=VERTEX_POINT('',#36821);
#11047=VERTEX_POINT('',#36823);
#11048=VERTEX_POINT('',#36827);
#11049=VERTEX_POINT('',#36831);
#11050=VERTEX_POINT('',#36835);
#11051=VERTEX_POINT('',#36840);
#11052=VERTEX_POINT('',#36846);
#11053=VERTEX_POINT('',#36850);
#11054=VERTEX_POINT('',#36854);
#11055=VERTEX_POINT('',#36860);
#11056=VERTEX_POINT('',#36861);
#11057=VERTEX_POINT('',#36863);
#11058=VERTEX_POINT('',#36867);
#11059=VERTEX_POINT('',#36868);
#11060=VERTEX_POINT('',#36870);
#11061=VERTEX_POINT('',#36874);
#11062=VERTEX_POINT('',#36875);
#11063=VERTEX_POINT('',#36880);
#11064=VERTEX_POINT('',#36881);
#11065=VERTEX_POINT('',#36886);
#11066=VERTEX_POINT('',#36887);
#11067=VERTEX_POINT('',#36892);
#11068=VERTEX_POINT('',#36893);
#11069=VERTEX_POINT('',#36904);
#11070=VERTEX_POINT('',#36905);
#11071=VERTEX_POINT('',#36908);
#11072=VERTEX_POINT('',#36912);
#11073=VERTEX_POINT('',#36913);
#11074=VERTEX_POINT('',#36916);
#11075=VERTEX_POINT('',#36920);
#11076=VERTEX_POINT('',#36926);
#11077=VERTEX_POINT('',#36930);
#11078=VERTEX_POINT('',#36934);
#11079=VERTEX_POINT('',#36938);
#11080=VERTEX_POINT('',#36967);
#11081=VERTEX_POINT('',#36975);
#11082=VERTEX_POINT('',#36990);
#11083=VERTEX_POINT('',#37020);
#11084=VERTEX_POINT('',#37023);
#11085=VERTEX_POINT('',#37026);
#11086=VERTEX_POINT('',#37029);
#11087=VERTEX_POINT('',#37032);
#13315=EDGE_CURVE('',#10904,#10905,#6592,.T.);
#13316=EDGE_CURVE('',#10905,#10906,#5731,.T.);
#13317=EDGE_CURVE('',#10906,#10907,#6593,.T.);
#13318=EDGE_CURVE('',#10907,#10904,#5732,.T.);
#13319=EDGE_CURVE('',#10908,#10909,#6594,.T.);
#13320=EDGE_CURVE('',#10909,#10905,#6595,.T.);
#13321=EDGE_CURVE('',#10904,#10908,#6596,.T.);
#13322=EDGE_CURVE('',#10910,#10911,#6597,.T.);
#13323=EDGE_CURVE('',#10911,#10909,#5733,.T.);
#13324=EDGE_CURVE('',#10908,#10910,#5734,.T.);
#13325=EDGE_CURVE('',#10912,#10913,#6598,.T.);
#13326=EDGE_CURVE('',#10913,#10911,#6599,.T.);
#13327=EDGE_CURVE('',#10910,#10912,#6600,.T.);
#13328=EDGE_CURVE('',#10914,#10915,#6601,.T.);
#13329=EDGE_CURVE('',#10915,#10913,#5735,.T.);
#13330=EDGE_CURVE('',#10912,#10914,#5736,.T.);
#13331=EDGE_CURVE('',#10916,#10917,#6602,.T.);
#13332=EDGE_CURVE('',#10917,#10915,#6603,.T.);
#13333=EDGE_CURVE('',#10914,#10916,#6604,.T.);
#13334=EDGE_CURVE('',#10918,#10919,#6605,.T.);
#13335=EDGE_CURVE('',#10919,#10917,#5737,.T.);
#13336=EDGE_CURVE('',#10916,#10918,#5738,.T.);
#13337=EDGE_CURVE('',#10906,#10919,#6606,.T.);
#13338=EDGE_CURVE('',#10918,#10907,#6607,.T.);
#13339=EDGE_CURVE('',#10917,#10920,#6608,.T.);
#13340=EDGE_CURVE('',#10921,#10920,#6609,.T.);
#13341=EDGE_CURVE('',#10921,#10915,#6610,.T.);
#13342=EDGE_CURVE('',#10922,#10919,#6611,.T.);
#13343=EDGE_CURVE('',#10920,#10922,#5739,.T.);
#13344=EDGE_CURVE('',#10923,#10906,#6612,.T.);
#13345=EDGE_CURVE('',#10922,#10923,#6613,.T.);
#13346=EDGE_CURVE('',#10924,#10905,#6614,.T.);
#13347=EDGE_CURVE('',#10923,#10924,#5740,.T.);
#13348=EDGE_CURVE('',#10925,#10926,#5741,.T.);
#13349=EDGE_CURVE('',#10927,#10925,#6615,.T.);
#13350=EDGE_CURVE('',#10928,#10927,#5742,.T.);
#13351=EDGE_CURVE('',#10929,#10928,#6616,.T.);
#13352=EDGE_CURVE('',#10930,#10929,#5743,.T.);
#13353=EDGE_CURVE('',#10931,#10930,#6617,.T.);
#13354=EDGE_CURVE('',#10932,#10931,#5744,.T.);
#13355=EDGE_CURVE('',#10926,#10932,#6618,.T.);
#13356=EDGE_CURVE('',#10933,#10933,#5745,.T.);
#13357=EDGE_CURVE('',#10933,#10934,#6619,.T.);
#13358=EDGE_CURVE('',#10934,#10934,#5746,.T.);
#13359=EDGE_CURVE('',#10935,#10936,#5747,.T.);
#13360=EDGE_CURVE('',#10937,#10935,#6620,.T.);
#13361=EDGE_CURVE('',#10938,#10937,#5748,.T.);
#13362=EDGE_CURVE('',#10939,#10938,#6621,.T.);
#13363=EDGE_CURVE('',#10940,#10939,#5749,.T.);
#13364=EDGE_CURVE('',#10941,#10940,#6622,.T.);
#13365=EDGE_CURVE('',#10942,#10941,#5750,.T.);
#13366=EDGE_CURVE('',#10936,#10942,#6623,.T.);
#13367=EDGE_CURVE('',#10943,#10943,#5751,.T.);
#13368=EDGE_CURVE('',#10944,#10944,#5752,.T.);
#13369=EDGE_CURVE('',#10945,#10945,#5753,.T.);
#13370=EDGE_CURVE('',#10946,#10947,#6624,.T.);
#13371=EDGE_CURVE('',#10948,#10946,#6625,.T.);
#13372=EDGE_CURVE('',#10949,#10948,#6626,.T.);
#13373=EDGE_CURVE('',#10947,#10949,#6627,.T.);
#13374=EDGE_CURVE('',#10950,#10950,#5754,.T.);
#13375=EDGE_CURVE('',#10951,#10951,#5755,.T.);
#13376=EDGE_CURVE('',#10951,#10934,#6628,.T.);
#13377=EDGE_CURVE('',#10943,#10952,#6629,.T.);
#13378=EDGE_CURVE('',#10952,#10952,#5756,.T.);
#13379=EDGE_CURVE('',#10953,#10953,#5757,.T.);
#13380=EDGE_CURVE('',#10953,#10952,#6630,.T.);
#13381=EDGE_CURVE('',#10950,#10954,#6631,.T.);
#13382=EDGE_CURVE('',#10954,#10954,#5758,.T.);
#13383=EDGE_CURVE('',#10955,#10955,#5759,.T.);
#13384=EDGE_CURVE('',#10955,#10954,#6632,.T.);
#13385=EDGE_CURVE('',#10944,#10956,#6633,.T.);
#13386=EDGE_CURVE('',#10956,#10956,#5760,.T.);
#13387=EDGE_CURVE('',#10957,#10957,#5761,.T.);
#13388=EDGE_CURVE('',#10957,#10956,#6634,.T.);
#13389=EDGE_CURVE('',#10948,#10958,#6635,.T.);
#13390=EDGE_CURVE('',#10958,#10959,#6636,.T.);
#13391=EDGE_CURVE('',#10949,#10959,#6637,.T.);
#13392=EDGE_CURVE('',#10947,#10960,#6638,.T.);
#13393=EDGE_CURVE('',#10960,#10961,#6639,.T.);
#13394=EDGE_CURVE('',#10961,#10946,#6640,.T.);
#13395=EDGE_CURVE('',#10959,#10960,#6641,.T.);
#13396=EDGE_CURVE('',#10961,#10958,#6642,.T.);
#13397=EDGE_CURVE('',#10961,#10962,#6643,.T.);
#13398=EDGE_CURVE('',#10962,#10963,#6644,.T.);
#13399=EDGE_CURVE('',#10958,#10963,#6645,.T.);
#13400=EDGE_CURVE('',#10960,#10964,#6646,.T.);
#13401=EDGE_CURVE('',#10964,#10962,#6647,.T.);
#13402=EDGE_CURVE('',#10965,#10966,#1089,.T.);
#13403=EDGE_CURVE('',#10966,#10967,#6648,.T.);
#13404=EDGE_CURVE('',#10967,#10921,#6649,.T.);
#13405=EDGE_CURVE('',#10920,#10968,#6650,.T.);
#13406=EDGE_CURVE('',#10968,#10965,#6651,.T.);
#13407=EDGE_CURVE('',#10969,#10970,#6652,.T.);
#13408=EDGE_CURVE('',#10970,#10921,#5762,.T.);
#13409=EDGE_CURVE('',#10967,#10969,#5763,.T.);
#13410=EDGE_CURVE('',#10971,#10972,#6653,.T.);
#13411=EDGE_CURVE('',#10972,#10970,#6654,.T.);
#13412=EDGE_CURVE('',#10969,#10971,#6655,.T.);
#13413=EDGE_CURVE('',#10973,#10974,#6656,.T.);
#13414=EDGE_CURVE('',#10974,#10972,#5764,.T.);
#13415=EDGE_CURVE('',#10971,#10973,#5765,.T.);
#13416=EDGE_CURVE('',#10975,#10976,#1090,.T.);
#13417=EDGE_CURVE('',#10976,#10977,#6657,.T.);
#13418=EDGE_CURVE('',#10977,#10924,#6658,.T.);
#13419=EDGE_CURVE('',#10924,#10974,#6659,.T.);
#13420=EDGE_CURVE('',#10973,#10975,#6660,.T.);
#13421=EDGE_CURVE('',#10978,#10923,#6661,.T.);
#13422=EDGE_CURVE('',#10977,#10978,#5766,.T.);
#13423=EDGE_CURVE('',#10979,#10922,#6662,.T.);
#13424=EDGE_CURVE('',#10978,#10979,#6663,.T.);
#13425=EDGE_CURVE('',#10979,#10968,#5767,.T.);
#13426=EDGE_CURVE('',#10968,#10980,#6664,.T.);
#13427=EDGE_CURVE('',#10981,#10980,#6665,.T.);
#13428=EDGE_CURVE('',#10967,#10981,#6666,.T.);
#13429=EDGE_CURVE('',#10966,#10982,#5768,.T.);
#13430=EDGE_CURVE('',#10982,#10965,#5769,.T.);
#13431=EDGE_CURVE('',#10979,#10983,#6667,.T.);
#13432=EDGE_CURVE('',#10980,#10983,#5770,.T.);
#13433=EDGE_CURVE('',#10978,#10984,#6668,.T.);
#13434=EDGE_CURVE('',#10983,#10984,#6669,.T.);
#13435=EDGE_CURVE('',#10977,#10985,#6670,.T.);
#13436=EDGE_CURVE('',#10984,#10985,#5771,.T.);
#13437=EDGE_CURVE('',#10976,#10986,#5772,.T.);
#13438=EDGE_CURVE('',#10986,#10975,#5773,.T.);
#13439=EDGE_CURVE('',#10973,#10987,#6671,.T.);
#13440=EDGE_CURVE('',#10985,#10987,#6672,.T.);
#13441=EDGE_CURVE('',#10986,#10988,#6673,.T.);
#13442=EDGE_CURVE('',#10989,#10988,#5774,.T.);
#13443=EDGE_CURVE('',#10990,#10989,#1091,.T.);
#13444=EDGE_CURVE('',#10988,#10990,#5775,.T.);
#13445=EDGE_CURVE('',#10991,#10992,#6674,.T.);
#13446=EDGE_CURVE('',#10992,#10993,#6675,.T.);
#13447=EDGE_CURVE('',#10993,#10994,#6676,.T.);
#13448=EDGE_CURVE('',#10994,#10995,#6677,.T.);
#13449=EDGE_CURVE('',#10995,#10991,#6678,.T.);
#13450=EDGE_CURVE('',#10995,#10996,#6679,.T.);
#13451=EDGE_CURVE('',#10996,#10997,#6680,.F.);
#13452=EDGE_CURVE('',#10997,#10991,#6681,.T.);
#13453=EDGE_CURVE('',#10992,#10998,#6682,.T.);
#13454=EDGE_CURVE('',#10998,#10999,#6683,.T.);
#13455=EDGE_CURVE('',#10999,#11000,#6684,.T.);
#13456=EDGE_CURVE('',#10993,#11000,#6685,.T.);
#13457=EDGE_CURVE('',#11001,#10997,#6686,.T.);
#13458=EDGE_CURVE('',#11002,#11001,#6687,.T.);
#13459=EDGE_CURVE('',#11002,#11003,#6688,.T.);
#13460=EDGE_CURVE('',#11004,#11003,#6689,.T.);
#13461=EDGE_CURVE('',#10998,#11004,#6690,.T.);
#13462=EDGE_CURVE('',#11000,#11005,#6691,.T.);
#13463=EDGE_CURVE('',#11005,#11006,#6692,.T.);
#13464=EDGE_CURVE('',#11006,#11007,#6693,.T.);
#13465=EDGE_CURVE('',#11007,#10994,#6694,.T.);
#13466=EDGE_CURVE('',#11008,#11006,#6695,.T.);
#13467=EDGE_CURVE('',#11008,#11009,#6696,.T.);
#13468=EDGE_CURVE('',#11009,#11010,#6697,.T.);
#13469=EDGE_CURVE('',#11010,#11007,#6698,.T.);
#13470=EDGE_CURVE('',#11005,#11011,#6699,.T.);
#13471=EDGE_CURVE('',#11012,#11011,#6700,.T.);
#13472=EDGE_CURVE('',#11012,#11008,#6701,.T.);
#13473=EDGE_CURVE('',#11013,#11000,#6702,.T.);
#13474=EDGE_CURVE('',#11014,#11013,#6703,.T.);
#13475=EDGE_CURVE('',#11005,#11014,#6704,.T.);
#13476=EDGE_CURVE('',#11015,#11014,#6705,.T.);
#13477=EDGE_CURVE('',#11013,#11016,#6706,.T.);
#13478=EDGE_CURVE('',#11016,#11015,#6707,.T.);
#13479=EDGE_CURVE('',#11015,#11017,#6708,.T.);
#13480=EDGE_CURVE('',#11017,#11011,#6709,.T.);
#13481=EDGE_CURVE('',#10926,#11018,#6710,.T.);
#13482=EDGE_CURVE('',#11018,#11019,#5776,.T.);
#13483=EDGE_CURVE('',#11019,#10925,#6711,.T.);
#13484=EDGE_CURVE('',#10932,#11020,#6712,.T.);
#13485=EDGE_CURVE('',#11020,#11018,#6713,.T.);
#13486=EDGE_CURVE('',#10931,#11021,#6714,.T.);
#13487=EDGE_CURVE('',#11021,#11020,#5777,.T.);
#13488=EDGE_CURVE('',#10930,#11022,#6715,.T.);
#13489=EDGE_CURVE('',#11022,#11021,#6716,.T.);
#13490=EDGE_CURVE('',#10929,#11023,#6717,.T.);
#13491=EDGE_CURVE('',#11023,#11022,#5778,.T.);
#13492=EDGE_CURVE('',#10928,#11024,#6718,.T.);
#13493=EDGE_CURVE('',#11024,#11023,#6719,.T.);
#13494=EDGE_CURVE('',#10927,#11025,#6720,.T.);
#13495=EDGE_CURVE('',#11025,#11024,#5779,.T.);
#13496=EDGE_CURVE('',#11019,#11025,#6721,.T.);
#13497=EDGE_CURVE('',#11024,#11026,#6722,.T.);
#13498=EDGE_CURVE('',#11027,#11026,#6723,.T.);
#13499=EDGE_CURVE('',#11027,#11023,#6724,.T.);
#13500=EDGE_CURVE('',#11028,#11025,#6725,.T.);
#13501=EDGE_CURVE('',#11026,#11028,#5780,.T.);
#13502=EDGE_CURVE('',#11029,#11019,#6726,.T.);
#13503=EDGE_CURVE('',#11028,#11029,#6727,.T.);
#13504=EDGE_CURVE('',#11030,#11018,#6728,.T.);
#13505=EDGE_CURVE('',#11029,#11030,#5781,.T.);
#13506=EDGE_CURVE('',#11031,#11027,#6729,.T.);
#13507=EDGE_CURVE('',#11026,#11032,#6730,.T.);
#13508=EDGE_CURVE('',#11032,#11031,#6731,.T.);
#13509=EDGE_CURVE('',#11033,#11034,#6732,.T.);
#13510=EDGE_CURVE('',#11034,#11027,#5782,.T.);
#13511=EDGE_CURVE('',#11031,#11033,#5783,.T.);
#13512=EDGE_CURVE('',#11035,#11036,#1092,.T.);
#13513=EDGE_CURVE('',#11036,#11037,#6733,.T.);
#13514=EDGE_CURVE('',#11037,#11038,#6734,.T.);
#13515=EDGE_CURVE('',#11038,#11034,#6735,.T.);
#13516=EDGE_CURVE('',#11033,#11035,#6736,.T.);
#13517=EDGE_CURVE('',#11004,#11039,#6737,.T.);
#13518=EDGE_CURVE('',#11039,#11038,#5784,.T.);
#13519=EDGE_CURVE('',#11037,#11004,#5785,.T.);
#13520=EDGE_CURVE('',#11003,#11030,#6738,.T.);
#13521=EDGE_CURVE('',#11030,#11039,#6739,.T.);
#13522=EDGE_CURVE('',#11040,#11029,#6740,.T.);
#13523=EDGE_CURVE('',#11003,#11040,#5786,.T.);
#13524=EDGE_CURVE('',#10989,#11041,#6741,.T.);
#13525=EDGE_CURVE('',#11041,#11028,#6742,.T.);
#13526=EDGE_CURVE('',#11040,#10990,#6743,.T.);
#13527=EDGE_CURVE('',#11041,#11032,#5787,.T.);
#13528=EDGE_CURVE('',#11042,#11033,#6744,.T.);
#13529=EDGE_CURVE('',#11043,#11042,#6745,.T.);
#13530=EDGE_CURVE('',#11043,#11037,#6746,.T.);
#13531=EDGE_CURVE('',#11036,#11044,#5788,.T.);
#13532=EDGE_CURVE('',#11044,#11035,#5789,.T.);
#13533=EDGE_CURVE('',#11012,#11031,#6747,.T.);
#13534=EDGE_CURVE('',#11042,#11012,#5790,.T.);
#13535=EDGE_CURVE('',#11045,#11032,#6748,.T.);
#13536=EDGE_CURVE('',#11046,#11045,#6749,.T.);
#13537=EDGE_CURVE('',#11047,#11046,#6750,.T.);
#13538=EDGE_CURVE('',#11009,#11047,#6751,.T.);
#13539=EDGE_CURVE('',#11048,#11041,#6752,.T.);
#13540=EDGE_CURVE('',#11045,#11048,#5791,.T.);
#13541=EDGE_CURVE('',#11049,#11040,#6753,.T.);
#13542=EDGE_CURVE('',#11048,#11049,#6754,.T.);
#13543=EDGE_CURVE('',#11043,#11050,#6755,.T.);
#13544=EDGE_CURVE('',#11050,#10999,#5792,.T.);
#13545=EDGE_CURVE('',#10998,#11043,#5793,.T.);
#13546=EDGE_CURVE('',#11042,#11051,#6756,.T.);
#13547=EDGE_CURVE('',#11051,#11050,#6757,.T.);
#13548=EDGE_CURVE('',#11011,#11051,#5794,.T.);
#13549=EDGE_CURVE('',#11052,#10999,#6758,.T.);
#13550=EDGE_CURVE('',#11052,#11016,#6759,.T.);
#13551=EDGE_CURVE('',#11053,#11050,#6760,.T.);
#13552=EDGE_CURVE('',#11053,#11052,#5795,.T.);
#13553=EDGE_CURVE('',#11054,#11051,#6761,.T.);
#13554=EDGE_CURVE('',#11054,#11053,#6762,.T.);
#13555=EDGE_CURVE('',#11017,#11054,#5796,.T.);
#13556=EDGE_CURVE('',#11055,#11056,#6763,.T.);
#13557=EDGE_CURVE('',#11057,#11055,#6764,.T.);
#13558=EDGE_CURVE('',#11056,#11057,#6765,.T.);
#13559=EDGE_CURVE('',#11058,#11059,#6766,.T.);
#13560=EDGE_CURVE('',#11060,#11058,#6767,.T.);
#13561=EDGE_CURVE('',#11059,#11060,#6768,.T.);
#13562=EDGE_CURVE('',#11061,#11062,#6769,.T.);
#13563=EDGE_CURVE('',#11062,#11057,#6770,.T.);
#13564=EDGE_CURVE('',#11055,#11061,#6771,.T.);
#13565=EDGE_CURVE('',#11063,#11064,#6772,.T.);
#13566=EDGE_CURVE('',#11064,#11062,#5797,.T.);
#13567=EDGE_CURVE('',#11061,#11063,#5798,.T.);
#13568=EDGE_CURVE('',#11065,#11066,#6773,.T.);
#13569=EDGE_CURVE('',#11066,#11064,#6774,.T.);
#13570=EDGE_CURVE('',#11063,#11065,#6775,.T.);
#13571=EDGE_CURVE('',#11067,#11068,#6776,.T.);
#13572=EDGE_CURVE('',#11068,#11066,#5799,.T.);
#13573=EDGE_CURVE('',#11065,#11067,#5800,.T.);
#13574=EDGE_CURVE('',#11067,#11060,#6777,.T.);
#13575=EDGE_CURVE('',#11058,#11068,#6778,.T.);
#13576=EDGE_CURVE('',#11056,#11059,#6779,.T.);
#13577=EDGE_CURVE('',#11060,#11055,#6780,.T.);
#13578=EDGE_CURVE('',#11069,#11070,#6781,.F.);
#13579=EDGE_CURVE('',#11001,#11069,#6782,.F.);
#13580=EDGE_CURVE('',#11071,#11001,#6783,.F.);
#13581=EDGE_CURVE('',#11070,#11071,#6784,.F.);
#13582=EDGE_CURVE('',#11072,#11073,#6785,.F.);
#13583=EDGE_CURVE('',#11046,#11072,#6786,.F.);
#13584=EDGE_CURVE('',#11074,#11046,#6787,.F.);
#13585=EDGE_CURVE('',#11073,#11074,#6788,.F.);
#13586=EDGE_CURVE('',#11072,#11075,#6789,.T.);
#13587=EDGE_CURVE('',#11075,#11047,#6790,.T.);
#13588=EDGE_CURVE('',#11075,#11010,#6791,.T.);
#13589=EDGE_CURVE('',#11045,#11076,#6792,.T.);
#13590=EDGE_CURVE('',#11076,#11074,#6793,.T.);
#13591=EDGE_CURVE('',#11048,#11077,#6794,.T.);
#13592=EDGE_CURVE('',#11077,#11076,#5801,.T.);
#13593=EDGE_CURVE('',#11049,#11078,#6795,.T.);
#13594=EDGE_CURVE('',#11078,#11077,#6796,.T.);
#13595=EDGE_CURVE('',#11002,#11079,#6797,.T.);
#13596=EDGE_CURVE('',#11079,#11078,#5802,.T.);
#13597=EDGE_CURVE('',#11049,#11002,#5803,.T.);
#13598=EDGE_CURVE('',#11069,#11079,#6798,.T.);
#13599=EDGE_CURVE('',#11059,#11073,#6799,.T.);
#13600=EDGE_CURVE('',#11074,#11058,#6800,.T.);
#13601=EDGE_CURVE('',#11073,#11070,#6801,.T.);
#13602=EDGE_CURVE('',#11071,#11072,#6802,.T.);
#13603=EDGE_CURVE('',#10996,#11071,#6803,.T.);
#13604=EDGE_CURVE('',#11057,#11069,#6804,.T.);
#13605=EDGE_CURVE('',#11070,#11056,#6805,.T.);
#13606=EDGE_CURVE('',#11064,#11078,#6806,.T.);
#13607=EDGE_CURVE('',#11062,#11079,#6807,.T.);
#13608=EDGE_CURVE('',#11068,#11076,#6808,.T.);
#13609=EDGE_CURVE('',#11066,#11077,#6809,.T.);
#13610=EDGE_CURVE('',#11010,#10995,#6810,.T.);
#13611=EDGE_CURVE('',#10996,#11075,#6811,.T.);
#13612=EDGE_CURVE('',#11080,#11080,#5804,.T.);
#13613=EDGE_CURVE('',#11081,#10935,#5805,.T.);
#13614=EDGE_CURVE('',#10936,#10987,#5806,.T.);
#13615=EDGE_CURVE('',#10987,#11081,#5807,.T.);
#13616=EDGE_CURVE('',#10942,#10985,#5808,.T.);
#13617=EDGE_CURVE('',#10941,#10984,#5809,.T.);
#13618=EDGE_CURVE('',#10940,#10983,#5810,.T.);
#13619=EDGE_CURVE('',#10939,#10980,#5811,.T.);
#13620=EDGE_CURVE('',#10938,#10981,#5812,.T.);
#13621=EDGE_CURVE('',#10937,#11082,#5813,.T.);
#13622=EDGE_CURVE('',#11082,#10981,#5814,.T.);
#13623=EDGE_CURVE('',#11081,#11082,#6812,.T.);
#13624=EDGE_CURVE('',#10969,#11082,#6813,.T.);
#13625=EDGE_CURVE('',#10971,#11081,#6814,.T.);
#13626=EDGE_CURVE('',#10970,#10913,#6815,.T.);
#13627=EDGE_CURVE('',#10972,#10911,#6816,.T.);
#13628=EDGE_CURVE('',#10974,#10909,#6817,.T.);
#13629=EDGE_CURVE('',#11034,#11022,#6818,.T.);
#13630=EDGE_CURVE('',#11038,#11021,#6819,.T.);
#13631=EDGE_CURVE('',#11039,#11020,#6820,.T.);
#13632=EDGE_CURVE('',#11044,#10982,#6821,.T.);
#13633=EDGE_CURVE('',#11080,#10945,#6822,.T.);
#13634=EDGE_CURVE('',#11083,#10951,#6823,.T.);
#13635=EDGE_CURVE('',#11084,#10953,#6824,.T.);
#13636=EDGE_CURVE('',#11085,#10955,#6825,.T.);
#13637=EDGE_CURVE('',#11086,#10957,#6826,.T.);
#13638=EDGE_CURVE('',#10959,#11087,#6827,.T.);
#13639=EDGE_CURVE('',#11087,#10964,#6828,.T.);
#13640=EDGE_CURVE('',#10963,#11087,#6829,.T.);
#17185=ORIENTED_EDGE('',*,*,#13315,.T.);
#17186=ORIENTED_EDGE('',*,*,#13316,.T.);
#17187=ORIENTED_EDGE('',*,*,#13317,.T.);
#17188=ORIENTED_EDGE('',*,*,#13318,.T.);
#17189=ORIENTED_EDGE('',*,*,#13319,.T.);
#17190=ORIENTED_EDGE('',*,*,#13320,.T.);
#17191=ORIENTED_EDGE('',*,*,#13315,.F.);
#17192=ORIENTED_EDGE('',*,*,#13321,.T.);
#17193=ORIENTED_EDGE('',*,*,#13322,.T.);
#17194=ORIENTED_EDGE('',*,*,#13323,.T.);
#17195=ORIENTED_EDGE('',*,*,#13319,.F.);
#17196=ORIENTED_EDGE('',*,*,#13324,.T.);
#17197=ORIENTED_EDGE('',*,*,#13325,.T.);
#17198=ORIENTED_EDGE('',*,*,#13326,.T.);
#17199=ORIENTED_EDGE('',*,*,#13322,.F.);
#17200=ORIENTED_EDGE('',*,*,#13327,.T.);
#17201=ORIENTED_EDGE('',*,*,#13328,.T.);
#17202=ORIENTED_EDGE('',*,*,#13329,.T.);
#17203=ORIENTED_EDGE('',*,*,#13325,.F.);
#17204=ORIENTED_EDGE('',*,*,#13330,.T.);
#17205=ORIENTED_EDGE('',*,*,#13331,.T.);
#17206=ORIENTED_EDGE('',*,*,#13332,.T.);
#17207=ORIENTED_EDGE('',*,*,#13328,.F.);
#17208=ORIENTED_EDGE('',*,*,#13333,.T.);
#17209=ORIENTED_EDGE('',*,*,#13334,.T.);
#17210=ORIENTED_EDGE('',*,*,#13335,.T.);
#17211=ORIENTED_EDGE('',*,*,#13331,.F.);
#17212=ORIENTED_EDGE('',*,*,#13336,.T.);
#17213=ORIENTED_EDGE('',*,*,#13317,.F.);
#17214=ORIENTED_EDGE('',*,*,#13337,.T.);
#17215=ORIENTED_EDGE('',*,*,#13334,.F.);
#17216=ORIENTED_EDGE('',*,*,#13338,.T.);
#17217=ORIENTED_EDGE('',*,*,#13332,.F.);
#17218=ORIENTED_EDGE('',*,*,#13339,.T.);
#17219=ORIENTED_EDGE('',*,*,#13340,.F.);
#17220=ORIENTED_EDGE('',*,*,#13341,.T.);
#17221=ORIENTED_EDGE('',*,*,#13335,.F.);
#17222=ORIENTED_EDGE('',*,*,#13342,.F.);
#17223=ORIENTED_EDGE('',*,*,#13343,.F.);
#17224=ORIENTED_EDGE('',*,*,#13339,.F.);
#17225=ORIENTED_EDGE('',*,*,#13337,.F.);
#17226=ORIENTED_EDGE('',*,*,#13344,.F.);
#17227=ORIENTED_EDGE('',*,*,#13345,.F.);
#17228=ORIENTED_EDGE('',*,*,#13342,.T.);
#17229=ORIENTED_EDGE('',*,*,#13316,.F.);
#17230=ORIENTED_EDGE('',*,*,#13346,.F.);
#17231=ORIENTED_EDGE('',*,*,#13347,.F.);
#17232=ORIENTED_EDGE('',*,*,#13344,.T.);
#17233=ORIENTED_EDGE('',*,*,#13348,.F.);
#17234=ORIENTED_EDGE('',*,*,#13349,.F.);
#17235=ORIENTED_EDGE('',*,*,#13350,.F.);
#17236=ORIENTED_EDGE('',*,*,#13351,.F.);
#17237=ORIENTED_EDGE('',*,*,#13352,.F.);
#17238=ORIENTED_EDGE('',*,*,#13353,.F.);
#17239=ORIENTED_EDGE('',*,*,#13354,.F.);
#17240=ORIENTED_EDGE('',*,*,#13355,.F.);
#17241=ORIENTED_EDGE('',*,*,#13318,.F.);
#17242=ORIENTED_EDGE('',*,*,#13338,.F.);
#17243=ORIENTED_EDGE('',*,*,#13336,.F.);
#17244=ORIENTED_EDGE('',*,*,#13333,.F.);
#17245=ORIENTED_EDGE('',*,*,#13330,.F.);
#17246=ORIENTED_EDGE('',*,*,#13327,.F.);
#17247=ORIENTED_EDGE('',*,*,#13324,.F.);
#17248=ORIENTED_EDGE('',*,*,#13321,.F.);
#17249=ORIENTED_EDGE('',*,*,#13356,.T.);
#17250=ORIENTED_EDGE('',*,*,#13357,.T.);
#17251=ORIENTED_EDGE('',*,*,#13358,.T.);
#17252=ORIENTED_EDGE('',*,*,#13357,.F.);
#17253=ORIENTED_EDGE('',*,*,#13359,.F.);
#17254=ORIENTED_EDGE('',*,*,#13360,.F.);
#17255=ORIENTED_EDGE('',*,*,#13361,.F.);
#17256=ORIENTED_EDGE('',*,*,#13362,.F.);
#17257=ORIENTED_EDGE('',*,*,#13363,.F.);
#17258=ORIENTED_EDGE('',*,*,#13364,.F.);
#17259=ORIENTED_EDGE('',*,*,#13365,.F.);
#17260=ORIENTED_EDGE('',*,*,#13366,.F.);
#17261=ORIENTED_EDGE('',*,*,#13367,.F.);
#17262=ORIENTED_EDGE('',*,*,#13368,.F.);
#17263=ORIENTED_EDGE('',*,*,#13369,.T.);
#17264=ORIENTED_EDGE('',*,*,#13370,.F.);
#17265=ORIENTED_EDGE('',*,*,#13371,.F.);
#17266=ORIENTED_EDGE('',*,*,#13372,.F.);
#17267=ORIENTED_EDGE('',*,*,#13373,.F.);
#17268=ORIENTED_EDGE('',*,*,#13374,.F.);
#17269=ORIENTED_EDGE('',*,*,#13356,.F.);
#17270=ORIENTED_EDGE('',*,*,#13375,.F.);
#17271=ORIENTED_EDGE('',*,*,#13376,.T.);
#17272=ORIENTED_EDGE('',*,*,#13358,.F.);
#17273=ORIENTED_EDGE('',*,*,#13376,.F.);
#17274=ORIENTED_EDGE('',*,*,#13367,.T.);
#17275=ORIENTED_EDGE('',*,*,#13377,.T.);
#17276=ORIENTED_EDGE('',*,*,#13378,.T.);
#17277=ORIENTED_EDGE('',*,*,#13377,.F.);
#17278=ORIENTED_EDGE('',*,*,#13379,.F.);
#17279=ORIENTED_EDGE('',*,*,#13380,.T.);
#17280=ORIENTED_EDGE('',*,*,#13378,.F.);
#17281=ORIENTED_EDGE('',*,*,#13380,.F.);
#17282=ORIENTED_EDGE('',*,*,#13374,.T.);
#17283=ORIENTED_EDGE('',*,*,#13381,.T.);
#17284=ORIENTED_EDGE('',*,*,#13382,.T.);
#17285=ORIENTED_EDGE('',*,*,#13381,.F.);
#17286=ORIENTED_EDGE('',*,*,#13383,.F.);
#17287=ORIENTED_EDGE('',*,*,#13384,.T.);
#17288=ORIENTED_EDGE('',*,*,#13382,.F.);
#17289=ORIENTED_EDGE('',*,*,#13384,.F.);
#17290=ORIENTED_EDGE('',*,*,#13368,.T.);
#17291=ORIENTED_EDGE('',*,*,#13385,.T.);
#17292=ORIENTED_EDGE('',*,*,#13386,.T.);
#17293=ORIENTED_EDGE('',*,*,#13385,.F.);
#17294=ORIENTED_EDGE('',*,*,#13387,.F.);
#17295=ORIENTED_EDGE('',*,*,#13388,.T.);
#17296=ORIENTED_EDGE('',*,*,#13386,.F.);
#17297=ORIENTED_EDGE('',*,*,#13388,.F.);
#17298=ORIENTED_EDGE('',*,*,#13372,.T.);
#17299=ORIENTED_EDGE('',*,*,#13389,.T.);
#17300=ORIENTED_EDGE('',*,*,#13390,.T.);
#17301=ORIENTED_EDGE('',*,*,#13391,.F.);
#17302=ORIENTED_EDGE('',*,*,#13370,.T.);
#17303=ORIENTED_EDGE('',*,*,#13392,.T.);
#17304=ORIENTED_EDGE('',*,*,#13393,.T.);
#17305=ORIENTED_EDGE('',*,*,#13394,.T.);
#17306=ORIENTED_EDGE('',*,*,#13395,.T.);
#17307=ORIENTED_EDGE('',*,*,#13392,.F.);
#17308=ORIENTED_EDGE('',*,*,#13373,.T.);
#17309=ORIENTED_EDGE('',*,*,#13391,.T.);
#17310=ORIENTED_EDGE('',*,*,#13371,.T.);
#17311=ORIENTED_EDGE('',*,*,#13394,.F.);
#17312=ORIENTED_EDGE('',*,*,#13396,.T.);
#17313=ORIENTED_EDGE('',*,*,#13389,.F.);
#17314=ORIENTED_EDGE('',*,*,#13396,.F.);
#17315=ORIENTED_EDGE('',*,*,#13397,.T.);
#17316=ORIENTED_EDGE('',*,*,#13398,.T.);
#17317=ORIENTED_EDGE('',*,*,#13399,.F.);
#17318=ORIENTED_EDGE('',*,*,#13393,.F.);
#17319=ORIENTED_EDGE('',*,*,#13400,.T.);
#17320=ORIENTED_EDGE('',*,*,#13401,.T.);
#17321=ORIENTED_EDGE('',*,*,#13397,.F.);
#17322=ORIENTED_EDGE('',*,*,#13402,.T.);
#17323=ORIENTED_EDGE('',*,*,#13403,.T.);
#17324=ORIENTED_EDGE('',*,*,#13404,.T.);
#17325=ORIENTED_EDGE('',*,*,#13340,.T.);
#17326=ORIENTED_EDGE('',*,*,#13405,.T.);
#17327=ORIENTED_EDGE('',*,*,#13406,.T.);
#17328=ORIENTED_EDGE('',*,*,#13407,.T.);
#17329=ORIENTED_EDGE('',*,*,#13408,.T.);
#17330=ORIENTED_EDGE('',*,*,#13404,.F.);
#17331=ORIENTED_EDGE('',*,*,#13409,.T.);
#17332=ORIENTED_EDGE('',*,*,#13410,.T.);
#17333=ORIENTED_EDGE('',*,*,#13411,.T.);
#17334=ORIENTED_EDGE('',*,*,#13407,.F.);
#17335=ORIENTED_EDGE('',*,*,#13412,.T.);
#17336=ORIENTED_EDGE('',*,*,#13413,.T.);
#17337=ORIENTED_EDGE('',*,*,#13414,.T.);
#17338=ORIENTED_EDGE('',*,*,#13410,.F.);
#17339=ORIENTED_EDGE('',*,*,#13415,.T.);
#17340=ORIENTED_EDGE('',*,*,#13416,.T.);
#17341=ORIENTED_EDGE('',*,*,#13417,.T.);
#17342=ORIENTED_EDGE('',*,*,#13418,.T.);
#17343=ORIENTED_EDGE('',*,*,#13419,.T.);
#17344=ORIENTED_EDGE('',*,*,#13413,.F.);
#17345=ORIENTED_EDGE('',*,*,#13420,.T.);
#17346=ORIENTED_EDGE('',*,*,#13421,.T.);
#17347=ORIENTED_EDGE('',*,*,#13347,.T.);
#17348=ORIENTED_EDGE('',*,*,#13418,.F.);
#17349=ORIENTED_EDGE('',*,*,#13422,.T.);
#17350=ORIENTED_EDGE('',*,*,#13423,.T.);
#17351=ORIENTED_EDGE('',*,*,#13345,.T.);
#17352=ORIENTED_EDGE('',*,*,#13421,.F.);
#17353=ORIENTED_EDGE('',*,*,#13424,.T.);
#17354=ORIENTED_EDGE('',*,*,#13405,.F.);
#17355=ORIENTED_EDGE('',*,*,#13343,.T.);
#17356=ORIENTED_EDGE('',*,*,#13423,.F.);
#17357=ORIENTED_EDGE('',*,*,#13425,.T.);
#17358=ORIENTED_EDGE('',*,*,#13406,.F.);
#17359=ORIENTED_EDGE('',*,*,#13426,.T.);
#17360=ORIENTED_EDGE('',*,*,#13427,.F.);
#17361=ORIENTED_EDGE('',*,*,#13428,.F.);
#17362=ORIENTED_EDGE('',*,*,#13403,.F.);
#17363=ORIENTED_EDGE('',*,*,#13429,.T.);
#17364=ORIENTED_EDGE('',*,*,#13430,.T.);
#17365=ORIENTED_EDGE('',*,*,#13425,.F.);
#17366=ORIENTED_EDGE('',*,*,#13431,.T.);
#17367=ORIENTED_EDGE('',*,*,#13432,.F.);
#17368=ORIENTED_EDGE('',*,*,#13426,.F.);
#17369=ORIENTED_EDGE('',*,*,#13424,.F.);
#17370=ORIENTED_EDGE('',*,*,#13433,.T.);
#17371=ORIENTED_EDGE('',*,*,#13434,.F.);
#17372=ORIENTED_EDGE('',*,*,#13431,.F.);
#17373=ORIENTED_EDGE('',*,*,#13422,.F.);
#17374=ORIENTED_EDGE('',*,*,#13435,.T.);
#17375=ORIENTED_EDGE('',*,*,#13436,.F.);
#17376=ORIENTED_EDGE('',*,*,#13433,.F.);
#17377=ORIENTED_EDGE('',*,*,#13417,.F.);
#17378=ORIENTED_EDGE('',*,*,#13437,.T.);
#17379=ORIENTED_EDGE('',*,*,#13438,.T.);
#17380=ORIENTED_EDGE('',*,*,#13420,.F.);
#17381=ORIENTED_EDGE('',*,*,#13439,.T.);
#17382=ORIENTED_EDGE('',*,*,#13440,.F.);
#17383=ORIENTED_EDGE('',*,*,#13435,.F.);
#17384=ORIENTED_EDGE('',*,*,#13416,.F.);
#17385=ORIENTED_EDGE('',*,*,#13438,.F.);
#17386=ORIENTED_EDGE('',*,*,#13441,.T.);
#17387=ORIENTED_EDGE('',*,*,#13442,.F.);
#17388=ORIENTED_EDGE('',*,*,#13443,.F.);
#17389=ORIENTED_EDGE('',*,*,#13444,.F.);
#17390=ORIENTED_EDGE('',*,*,#13441,.F.);
#17391=ORIENTED_EDGE('',*,*,#13437,.F.);
#17392=ORIENTED_EDGE('',*,*,#13445,.T.);
#17393=ORIENTED_EDGE('',*,*,#13446,.T.);
#17394=ORIENTED_EDGE('',*,*,#13447,.T.);
#17395=ORIENTED_EDGE('',*,*,#13448,.T.);
#17396=ORIENTED_EDGE('',*,*,#13449,.T.);
#17397=ORIENTED_EDGE('',*,*,#13450,.T.);
#17398=ORIENTED_EDGE('',*,*,#13451,.T.);
#17399=ORIENTED_EDGE('',*,*,#13452,.T.);
#17400=ORIENTED_EDGE('',*,*,#13449,.F.);
#17401=ORIENTED_EDGE('',*,*,#13446,.F.);
#17402=ORIENTED_EDGE('',*,*,#13453,.T.);
#17403=ORIENTED_EDGE('',*,*,#13454,.T.);
#17404=ORIENTED_EDGE('',*,*,#13455,.T.);
#17405=ORIENTED_EDGE('',*,*,#13456,.F.);
#17406=ORIENTED_EDGE('',*,*,#13445,.F.);
#17407=ORIENTED_EDGE('',*,*,#13452,.F.);
#17408=ORIENTED_EDGE('',*,*,#13457,.F.);
#17409=ORIENTED_EDGE('',*,*,#13458,.F.);
#17410=ORIENTED_EDGE('',*,*,#13459,.T.);
#17411=ORIENTED_EDGE('',*,*,#13460,.F.);
#17412=ORIENTED_EDGE('',*,*,#13461,.F.);
#17413=ORIENTED_EDGE('',*,*,#13453,.F.);
#17414=ORIENTED_EDGE('',*,*,#13447,.F.);
#17415=ORIENTED_EDGE('',*,*,#13456,.T.);
#17416=ORIENTED_EDGE('',*,*,#13462,.T.);
#17417=ORIENTED_EDGE('',*,*,#13463,.T.);
#17418=ORIENTED_EDGE('',*,*,#13464,.T.);
#17419=ORIENTED_EDGE('',*,*,#13465,.T.);
#17420=ORIENTED_EDGE('',*,*,#13464,.F.);
#17421=ORIENTED_EDGE('',*,*,#13466,.F.);
#17422=ORIENTED_EDGE('',*,*,#13467,.T.);
#17423=ORIENTED_EDGE('',*,*,#13468,.T.);
#17424=ORIENTED_EDGE('',*,*,#13469,.T.);
#17425=ORIENTED_EDGE('',*,*,#13463,.F.);
#17426=ORIENTED_EDGE('',*,*,#13470,.T.);
#17427=ORIENTED_EDGE('',*,*,#13471,.F.);
#17428=ORIENTED_EDGE('',*,*,#13472,.T.);
#17429=ORIENTED_EDGE('',*,*,#13466,.T.);
#17430=ORIENTED_EDGE('',*,*,#13462,.F.);
#17431=ORIENTED_EDGE('',*,*,#13473,.F.);
#17432=ORIENTED_EDGE('',*,*,#13474,.F.);
#17433=ORIENTED_EDGE('',*,*,#13475,.F.);
#17434=ORIENTED_EDGE('',*,*,#13476,.T.);
#17435=ORIENTED_EDGE('',*,*,#13474,.T.);
#17436=ORIENTED_EDGE('',*,*,#13477,.T.);
#17437=ORIENTED_EDGE('',*,*,#13478,.T.);
#17438=ORIENTED_EDGE('',*,*,#13476,.F.);
#17439=ORIENTED_EDGE('',*,*,#13479,.T.);
#17440=ORIENTED_EDGE('',*,*,#13480,.T.);
#17441=ORIENTED_EDGE('',*,*,#13470,.F.);
#17442=ORIENTED_EDGE('',*,*,#13475,.T.);
#17443=ORIENTED_EDGE('',*,*,#13481,.T.);
#17444=ORIENTED_EDGE('',*,*,#13482,.T.);
#17445=ORIENTED_EDGE('',*,*,#13483,.T.);
#17446=ORIENTED_EDGE('',*,*,#13348,.T.);
#17447=ORIENTED_EDGE('',*,*,#13484,.T.);
#17448=ORIENTED_EDGE('',*,*,#13485,.T.);
#17449=ORIENTED_EDGE('',*,*,#13481,.F.);
#17450=ORIENTED_EDGE('',*,*,#13355,.T.);
#17451=ORIENTED_EDGE('',*,*,#13486,.T.);
#17452=ORIENTED_EDGE('',*,*,#13487,.T.);
#17453=ORIENTED_EDGE('',*,*,#13484,.F.);
#17454=ORIENTED_EDGE('',*,*,#13354,.T.);
#17455=ORIENTED_EDGE('',*,*,#13488,.T.);
#17456=ORIENTED_EDGE('',*,*,#13489,.T.);
#17457=ORIENTED_EDGE('',*,*,#13486,.F.);
#17458=ORIENTED_EDGE('',*,*,#13353,.T.);
#17459=ORIENTED_EDGE('',*,*,#13490,.T.);
#17460=ORIENTED_EDGE('',*,*,#13491,.T.);
#17461=ORIENTED_EDGE('',*,*,#13488,.F.);
#17462=ORIENTED_EDGE('',*,*,#13352,.T.);
#17463=ORIENTED_EDGE('',*,*,#13492,.T.);
#17464=ORIENTED_EDGE('',*,*,#13493,.T.);
#17465=ORIENTED_EDGE('',*,*,#13490,.F.);
#17466=ORIENTED_EDGE('',*,*,#13351,.T.);
#17467=ORIENTED_EDGE('',*,*,#13494,.T.);
#17468=ORIENTED_EDGE('',*,*,#13495,.T.);
#17469=ORIENTED_EDGE('',*,*,#13492,.F.);
#17470=ORIENTED_EDGE('',*,*,#13350,.T.);
#17471=ORIENTED_EDGE('',*,*,#13483,.F.);
#17472=ORIENTED_EDGE('',*,*,#13496,.T.);
#17473=ORIENTED_EDGE('',*,*,#13494,.F.);
#17474=ORIENTED_EDGE('',*,*,#13349,.T.);
#17475=ORIENTED_EDGE('',*,*,#13493,.F.);
#17476=ORIENTED_EDGE('',*,*,#13497,.T.);
#17477=ORIENTED_EDGE('',*,*,#13498,.F.);
#17478=ORIENTED_EDGE('',*,*,#13499,.T.);
#17479=ORIENTED_EDGE('',*,*,#13495,.F.);
#17480=ORIENTED_EDGE('',*,*,#13500,.F.);
#17481=ORIENTED_EDGE('',*,*,#13501,.F.);
#17482=ORIENTED_EDGE('',*,*,#13497,.F.);
#17483=ORIENTED_EDGE('',*,*,#13496,.F.);
#17484=ORIENTED_EDGE('',*,*,#13502,.F.);
#17485=ORIENTED_EDGE('',*,*,#13503,.F.);
#17486=ORIENTED_EDGE('',*,*,#13500,.T.);
#17487=ORIENTED_EDGE('',*,*,#13482,.F.);
#17488=ORIENTED_EDGE('',*,*,#13504,.F.);
#17489=ORIENTED_EDGE('',*,*,#13505,.F.);
#17490=ORIENTED_EDGE('',*,*,#13502,.T.);
#17491=ORIENTED_EDGE('',*,*,#13506,.T.);
#17492=ORIENTED_EDGE('',*,*,#13498,.T.);
#17493=ORIENTED_EDGE('',*,*,#13507,.T.);
#17494=ORIENTED_EDGE('',*,*,#13508,.T.);
#17495=ORIENTED_EDGE('',*,*,#13509,.T.);
#17496=ORIENTED_EDGE('',*,*,#13510,.T.);
#17497=ORIENTED_EDGE('',*,*,#13506,.F.);
#17498=ORIENTED_EDGE('',*,*,#13511,.T.);
#17499=ORIENTED_EDGE('',*,*,#13512,.T.);
#17500=ORIENTED_EDGE('',*,*,#13513,.T.);
#17501=ORIENTED_EDGE('',*,*,#13514,.T.);
#17502=ORIENTED_EDGE('',*,*,#13515,.T.);
#17503=ORIENTED_EDGE('',*,*,#13509,.F.);
#17504=ORIENTED_EDGE('',*,*,#13516,.T.);
#17505=ORIENTED_EDGE('',*,*,#13517,.T.);
#17506=ORIENTED_EDGE('',*,*,#13518,.T.);
#17507=ORIENTED_EDGE('',*,*,#13514,.F.);
#17508=ORIENTED_EDGE('',*,*,#13519,.T.);
#17509=ORIENTED_EDGE('',*,*,#13520,.T.);
#17510=ORIENTED_EDGE('',*,*,#13521,.T.);
#17511=ORIENTED_EDGE('',*,*,#13517,.F.);
#17512=ORIENTED_EDGE('',*,*,#13460,.T.);
#17513=ORIENTED_EDGE('',*,*,#13522,.T.);
#17514=ORIENTED_EDGE('',*,*,#13505,.T.);
#17515=ORIENTED_EDGE('',*,*,#13520,.F.);
#17516=ORIENTED_EDGE('',*,*,#13523,.T.);
#17517=ORIENTED_EDGE('',*,*,#13443,.T.);
#17518=ORIENTED_EDGE('',*,*,#13524,.T.);
#17519=ORIENTED_EDGE('',*,*,#13525,.T.);
#17520=ORIENTED_EDGE('',*,*,#13503,.T.);
#17521=ORIENTED_EDGE('',*,*,#13522,.F.);
#17522=ORIENTED_EDGE('',*,*,#13526,.T.);
#17523=ORIENTED_EDGE('',*,*,#13507,.F.);
#17524=ORIENTED_EDGE('',*,*,#13501,.T.);
#17525=ORIENTED_EDGE('',*,*,#13525,.F.);
#17526=ORIENTED_EDGE('',*,*,#13527,.T.);
#17527=ORIENTED_EDGE('',*,*,#13516,.F.);
#17528=ORIENTED_EDGE('',*,*,#13528,.F.);
#17529=ORIENTED_EDGE('',*,*,#13529,.F.);
#17530=ORIENTED_EDGE('',*,*,#13530,.T.);
#17531=ORIENTED_EDGE('',*,*,#13513,.F.);
#17532=ORIENTED_EDGE('',*,*,#13531,.T.);
#17533=ORIENTED_EDGE('',*,*,#13532,.T.);
#17534=ORIENTED_EDGE('',*,*,#13511,.F.);
#17535=ORIENTED_EDGE('',*,*,#13533,.F.);
#17536=ORIENTED_EDGE('',*,*,#13534,.F.);
#17537=ORIENTED_EDGE('',*,*,#13528,.T.);
#17538=ORIENTED_EDGE('',*,*,#13508,.F.);
#17539=ORIENTED_EDGE('',*,*,#13535,.F.);
#17540=ORIENTED_EDGE('',*,*,#13536,.F.);
#17541=ORIENTED_EDGE('',*,*,#13537,.F.);
#17542=ORIENTED_EDGE('',*,*,#13538,.F.);
#17543=ORIENTED_EDGE('',*,*,#13467,.F.);
#17544=ORIENTED_EDGE('',*,*,#13472,.F.);
#17545=ORIENTED_EDGE('',*,*,#13533,.T.);
#17546=ORIENTED_EDGE('',*,*,#13527,.F.);
#17547=ORIENTED_EDGE('',*,*,#13539,.F.);
#17548=ORIENTED_EDGE('',*,*,#13540,.F.);
#17549=ORIENTED_EDGE('',*,*,#13535,.T.);
#17550=ORIENTED_EDGE('',*,*,#13524,.F.);
#17551=ORIENTED_EDGE('',*,*,#13442,.T.);
#17552=ORIENTED_EDGE('',*,*,#13444,.T.);
#17553=ORIENTED_EDGE('',*,*,#13526,.F.);
#17554=ORIENTED_EDGE('',*,*,#13541,.F.);
#17555=ORIENTED_EDGE('',*,*,#13542,.F.);
#17556=ORIENTED_EDGE('',*,*,#13539,.T.);
#17557=ORIENTED_EDGE('',*,*,#13543,.T.);
#17558=ORIENTED_EDGE('',*,*,#13544,.T.);
#17559=ORIENTED_EDGE('',*,*,#13454,.F.);
#17560=ORIENTED_EDGE('',*,*,#13545,.T.);
#17561=ORIENTED_EDGE('',*,*,#13546,.T.);
#17562=ORIENTED_EDGE('',*,*,#13547,.T.);
#17563=ORIENTED_EDGE('',*,*,#13543,.F.);
#17564=ORIENTED_EDGE('',*,*,#13529,.T.);
#17565=ORIENTED_EDGE('',*,*,#13471,.T.);
#17566=ORIENTED_EDGE('',*,*,#13548,.T.);
#17567=ORIENTED_EDGE('',*,*,#13546,.F.);
#17568=ORIENTED_EDGE('',*,*,#13534,.T.);
#17569=ORIENTED_EDGE('',*,*,#13477,.F.);
#17570=ORIENTED_EDGE('',*,*,#13473,.T.);
#17571=ORIENTED_EDGE('',*,*,#13455,.F.);
#17572=ORIENTED_EDGE('',*,*,#13549,.F.);
#17573=ORIENTED_EDGE('',*,*,#13550,.T.);
#17574=ORIENTED_EDGE('',*,*,#13544,.F.);
#17575=ORIENTED_EDGE('',*,*,#13551,.F.);
#17576=ORIENTED_EDGE('',*,*,#13552,.T.);
#17577=ORIENTED_EDGE('',*,*,#13549,.T.);
#17578=ORIENTED_EDGE('',*,*,#13547,.F.);
#17579=ORIENTED_EDGE('',*,*,#13553,.F.);
#17580=ORIENTED_EDGE('',*,*,#13554,.T.);
#17581=ORIENTED_EDGE('',*,*,#13551,.T.);
#17582=ORIENTED_EDGE('',*,*,#13548,.F.);
#17583=ORIENTED_EDGE('',*,*,#13480,.F.);
#17584=ORIENTED_EDGE('',*,*,#13555,.T.);
#17585=ORIENTED_EDGE('',*,*,#13553,.T.);
#17586=ORIENTED_EDGE('',*,*,#13556,.F.);
#17587=ORIENTED_EDGE('',*,*,#13557,.F.);
#17588=ORIENTED_EDGE('',*,*,#13558,.F.);
#17589=ORIENTED_EDGE('',*,*,#13559,.F.);
#17590=ORIENTED_EDGE('',*,*,#13560,.F.);
#17591=ORIENTED_EDGE('',*,*,#13561,.F.);
#17592=ORIENTED_EDGE('',*,*,#13562,.T.);
#17593=ORIENTED_EDGE('',*,*,#13563,.T.);
#17594=ORIENTED_EDGE('',*,*,#13557,.T.);
#17595=ORIENTED_EDGE('',*,*,#13564,.T.);
#17596=ORIENTED_EDGE('',*,*,#13565,.T.);
#17597=ORIENTED_EDGE('',*,*,#13566,.T.);
#17598=ORIENTED_EDGE('',*,*,#13562,.F.);
#17599=ORIENTED_EDGE('',*,*,#13567,.T.);
#17600=ORIENTED_EDGE('',*,*,#13568,.T.);
#17601=ORIENTED_EDGE('',*,*,#13569,.T.);
#17602=ORIENTED_EDGE('',*,*,#13565,.F.);
#17603=ORIENTED_EDGE('',*,*,#13570,.T.);
#17604=ORIENTED_EDGE('',*,*,#13571,.T.);
#17605=ORIENTED_EDGE('',*,*,#13572,.T.);
#17606=ORIENTED_EDGE('',*,*,#13568,.F.);
#17607=ORIENTED_EDGE('',*,*,#13573,.T.);
#17608=ORIENTED_EDGE('',*,*,#13571,.F.);
#17609=ORIENTED_EDGE('',*,*,#13574,.T.);
#17610=ORIENTED_EDGE('',*,*,#13560,.T.);
#17611=ORIENTED_EDGE('',*,*,#13575,.T.);
#17612=ORIENTED_EDGE('',*,*,#13556,.T.);
#17613=ORIENTED_EDGE('',*,*,#13576,.T.);
#17614=ORIENTED_EDGE('',*,*,#13561,.T.);
#17615=ORIENTED_EDGE('',*,*,#13577,.T.);
#17616=ORIENTED_EDGE('',*,*,#13578,.F.);
#17617=ORIENTED_EDGE('',*,*,#13579,.F.);
#17618=ORIENTED_EDGE('',*,*,#13580,.F.);
#17619=ORIENTED_EDGE('',*,*,#13581,.F.);
#17620=ORIENTED_EDGE('',*,*,#13582,.F.);
#17621=ORIENTED_EDGE('',*,*,#13583,.F.);
#17622=ORIENTED_EDGE('',*,*,#13584,.F.);
#17623=ORIENTED_EDGE('',*,*,#13585,.F.);
#17624=ORIENTED_EDGE('',*,*,#13537,.T.);
#17625=ORIENTED_EDGE('',*,*,#13583,.T.);
#17626=ORIENTED_EDGE('',*,*,#13586,.T.);
#17627=ORIENTED_EDGE('',*,*,#13587,.T.);
#17628=ORIENTED_EDGE('',*,*,#13588,.T.);
#17629=ORIENTED_EDGE('',*,*,#13468,.F.);
#17630=ORIENTED_EDGE('',*,*,#13538,.T.);
#17631=ORIENTED_EDGE('',*,*,#13587,.F.);
#17632=ORIENTED_EDGE('',*,*,#13589,.T.);
#17633=ORIENTED_EDGE('',*,*,#13590,.T.);
#17634=ORIENTED_EDGE('',*,*,#13584,.T.);
#17635=ORIENTED_EDGE('',*,*,#13536,.T.);
#17636=ORIENTED_EDGE('',*,*,#13591,.T.);
#17637=ORIENTED_EDGE('',*,*,#13592,.T.);
#17638=ORIENTED_EDGE('',*,*,#13589,.F.);
#17639=ORIENTED_EDGE('',*,*,#13540,.T.);
#17640=ORIENTED_EDGE('',*,*,#13593,.T.);
#17641=ORIENTED_EDGE('',*,*,#13594,.T.);
#17642=ORIENTED_EDGE('',*,*,#13591,.F.);
#17643=ORIENTED_EDGE('',*,*,#13542,.T.);
#17644=ORIENTED_EDGE('',*,*,#13595,.T.);
#17645=ORIENTED_EDGE('',*,*,#13596,.T.);
#17646=ORIENTED_EDGE('',*,*,#13593,.F.);
#17647=ORIENTED_EDGE('',*,*,#13597,.T.);
#17648=ORIENTED_EDGE('',*,*,#13595,.F.);
#17649=ORIENTED_EDGE('',*,*,#13458,.T.);
#17650=ORIENTED_EDGE('',*,*,#13579,.T.);
#17651=ORIENTED_EDGE('',*,*,#13598,.T.);
#17652=ORIENTED_EDGE('',*,*,#13559,.T.);
#17653=ORIENTED_EDGE('',*,*,#13599,.T.);
#17654=ORIENTED_EDGE('',*,*,#13585,.T.);
#17655=ORIENTED_EDGE('',*,*,#13600,.T.);
#17656=ORIENTED_EDGE('',*,*,#13582,.T.);
#17657=ORIENTED_EDGE('',*,*,#13601,.T.);
#17658=ORIENTED_EDGE('',*,*,#13581,.T.);
#17659=ORIENTED_EDGE('',*,*,#13602,.T.);
#17660=ORIENTED_EDGE('',*,*,#13603,.T.);
#17661=ORIENTED_EDGE('',*,*,#13580,.T.);
#17662=ORIENTED_EDGE('',*,*,#13457,.T.);
#17663=ORIENTED_EDGE('',*,*,#13451,.F.);
#17664=ORIENTED_EDGE('',*,*,#13558,.T.);
#17665=ORIENTED_EDGE('',*,*,#13604,.T.);
#17666=ORIENTED_EDGE('',*,*,#13578,.T.);
#17667=ORIENTED_EDGE('',*,*,#13605,.T.);
#17668=ORIENTED_EDGE('',*,*,#13566,.F.);
#17669=ORIENTED_EDGE('',*,*,#13606,.T.);
#17670=ORIENTED_EDGE('',*,*,#13596,.F.);
#17671=ORIENTED_EDGE('',*,*,#13607,.F.);
#17672=ORIENTED_EDGE('',*,*,#13575,.F.);
#17673=ORIENTED_EDGE('',*,*,#13600,.F.);
#17674=ORIENTED_EDGE('',*,*,#13590,.F.);
#17675=ORIENTED_EDGE('',*,*,#13608,.F.);
#17676=ORIENTED_EDGE('',*,*,#13569,.F.);
#17677=ORIENTED_EDGE('',*,*,#13609,.T.);
#17678=ORIENTED_EDGE('',*,*,#13594,.F.);
#17679=ORIENTED_EDGE('',*,*,#13606,.F.);
#17680=ORIENTED_EDGE('',*,*,#13572,.F.);
#17681=ORIENTED_EDGE('',*,*,#13608,.T.);
#17682=ORIENTED_EDGE('',*,*,#13592,.F.);
#17683=ORIENTED_EDGE('',*,*,#13609,.F.);
#17684=ORIENTED_EDGE('',*,*,#13448,.F.);
#17685=ORIENTED_EDGE('',*,*,#13465,.F.);
#17686=ORIENTED_EDGE('',*,*,#13469,.F.);
#17687=ORIENTED_EDGE('',*,*,#13610,.T.);
#17688=ORIENTED_EDGE('',*,*,#13450,.F.);
#17689=ORIENTED_EDGE('',*,*,#13610,.F.);
#17690=ORIENTED_EDGE('',*,*,#13588,.F.);
#17691=ORIENTED_EDGE('',*,*,#13611,.F.);
#17692=ORIENTED_EDGE('',*,*,#13612,.T.);
#17693=ORIENTED_EDGE('',*,*,#13586,.F.);
#17694=ORIENTED_EDGE('',*,*,#13602,.F.);
#17695=ORIENTED_EDGE('',*,*,#13603,.F.);
#17696=ORIENTED_EDGE('',*,*,#13611,.T.);
#17697=ORIENTED_EDGE('',*,*,#13564,.F.);
#17698=ORIENTED_EDGE('',*,*,#13577,.F.);
#17699=ORIENTED_EDGE('',*,*,#13574,.F.);
#17700=ORIENTED_EDGE('',*,*,#13573,.F.);
#17701=ORIENTED_EDGE('',*,*,#13570,.F.);
#17702=ORIENTED_EDGE('',*,*,#13567,.F.);
#17703=ORIENTED_EDGE('',*,*,#13576,.F.);
#17704=ORIENTED_EDGE('',*,*,#13605,.F.);
#17705=ORIENTED_EDGE('',*,*,#13601,.F.);
#17706=ORIENTED_EDGE('',*,*,#13599,.F.);
#17707=ORIENTED_EDGE('',*,*,#13563,.F.);
#17708=ORIENTED_EDGE('',*,*,#13607,.T.);
#17709=ORIENTED_EDGE('',*,*,#13598,.F.);
#17710=ORIENTED_EDGE('',*,*,#13604,.F.);
#17711=ORIENTED_EDGE('',*,*,#13478,.F.);
#17712=ORIENTED_EDGE('',*,*,#13550,.F.);
#17713=ORIENTED_EDGE('',*,*,#13552,.F.);
#17714=ORIENTED_EDGE('',*,*,#13554,.F.);
#17715=ORIENTED_EDGE('',*,*,#13555,.F.);
#17716=ORIENTED_EDGE('',*,*,#13479,.F.);
#17717=ORIENTED_EDGE('',*,*,#13613,.T.);
#17718=ORIENTED_EDGE('',*,*,#13359,.T.);
#17719=ORIENTED_EDGE('',*,*,#13614,.T.);
#17720=ORIENTED_EDGE('',*,*,#13615,.T.);
#17721=ORIENTED_EDGE('',*,*,#13616,.T.);
#17722=ORIENTED_EDGE('',*,*,#13440,.T.);
#17723=ORIENTED_EDGE('',*,*,#13614,.F.);
#17724=ORIENTED_EDGE('',*,*,#13366,.T.);
#17725=ORIENTED_EDGE('',*,*,#13617,.T.);
#17726=ORIENTED_EDGE('',*,*,#13436,.T.);
#17727=ORIENTED_EDGE('',*,*,#13616,.F.);
#17728=ORIENTED_EDGE('',*,*,#13365,.T.);
#17729=ORIENTED_EDGE('',*,*,#13618,.T.);
#17730=ORIENTED_EDGE('',*,*,#13434,.T.);
#17731=ORIENTED_EDGE('',*,*,#13617,.F.);
#17732=ORIENTED_EDGE('',*,*,#13364,.T.);
#17733=ORIENTED_EDGE('',*,*,#13619,.T.);
#17734=ORIENTED_EDGE('',*,*,#13432,.T.);
#17735=ORIENTED_EDGE('',*,*,#13618,.F.);
#17736=ORIENTED_EDGE('',*,*,#13363,.T.);
#17737=ORIENTED_EDGE('',*,*,#13620,.T.);
#17738=ORIENTED_EDGE('',*,*,#13427,.T.);
#17739=ORIENTED_EDGE('',*,*,#13619,.F.);
#17740=ORIENTED_EDGE('',*,*,#13362,.T.);
#17741=ORIENTED_EDGE('',*,*,#13621,.T.);
#17742=ORIENTED_EDGE('',*,*,#13622,.T.);
#17743=ORIENTED_EDGE('',*,*,#13620,.F.);
#17744=ORIENTED_EDGE('',*,*,#13361,.T.);
#17745=ORIENTED_EDGE('',*,*,#13613,.F.);
#17746=ORIENTED_EDGE('',*,*,#13623,.T.);
#17747=ORIENTED_EDGE('',*,*,#13621,.F.);
#17748=ORIENTED_EDGE('',*,*,#13360,.T.);
#17749=ORIENTED_EDGE('',*,*,#13409,.F.);
#17750=ORIENTED_EDGE('',*,*,#13428,.T.);
#17751=ORIENTED_EDGE('',*,*,#13622,.F.);
#17752=ORIENTED_EDGE('',*,*,#13624,.F.);
#17753=ORIENTED_EDGE('',*,*,#13412,.F.);
#17754=ORIENTED_EDGE('',*,*,#13624,.T.);
#17755=ORIENTED_EDGE('',*,*,#13623,.F.);
#17756=ORIENTED_EDGE('',*,*,#13625,.F.);
#17757=ORIENTED_EDGE('',*,*,#13415,.F.);
#17758=ORIENTED_EDGE('',*,*,#13625,.T.);
#17759=ORIENTED_EDGE('',*,*,#13615,.F.);
#17760=ORIENTED_EDGE('',*,*,#13439,.F.);
#17761=ORIENTED_EDGE('',*,*,#13329,.F.);
#17762=ORIENTED_EDGE('',*,*,#13341,.F.);
#17763=ORIENTED_EDGE('',*,*,#13408,.F.);
#17764=ORIENTED_EDGE('',*,*,#13626,.T.);
#17765=ORIENTED_EDGE('',*,*,#13326,.F.);
#17766=ORIENTED_EDGE('',*,*,#13626,.F.);
#17767=ORIENTED_EDGE('',*,*,#13411,.F.);
#17768=ORIENTED_EDGE('',*,*,#13627,.T.);
#17769=ORIENTED_EDGE('',*,*,#13323,.F.);
#17770=ORIENTED_EDGE('',*,*,#13627,.F.);
#17771=ORIENTED_EDGE('',*,*,#13414,.F.);
#17772=ORIENTED_EDGE('',*,*,#13628,.T.);
#17773=ORIENTED_EDGE('',*,*,#13320,.F.);
#17774=ORIENTED_EDGE('',*,*,#13628,.F.);
#17775=ORIENTED_EDGE('',*,*,#13419,.F.);
#17776=ORIENTED_EDGE('',*,*,#13346,.T.);
#17777=ORIENTED_EDGE('',*,*,#13491,.F.);
#17778=ORIENTED_EDGE('',*,*,#13499,.F.);
#17779=ORIENTED_EDGE('',*,*,#13510,.F.);
#17780=ORIENTED_EDGE('',*,*,#13629,.T.);
#17781=ORIENTED_EDGE('',*,*,#13489,.F.);
#17782=ORIENTED_EDGE('',*,*,#13629,.F.);
#17783=ORIENTED_EDGE('',*,*,#13515,.F.);
#17784=ORIENTED_EDGE('',*,*,#13630,.T.);
#17785=ORIENTED_EDGE('',*,*,#13487,.F.);
#17786=ORIENTED_EDGE('',*,*,#13630,.F.);
#17787=ORIENTED_EDGE('',*,*,#13518,.F.);
#17788=ORIENTED_EDGE('',*,*,#13631,.T.);
#17789=ORIENTED_EDGE('',*,*,#13485,.F.);
#17790=ORIENTED_EDGE('',*,*,#13631,.F.);
#17791=ORIENTED_EDGE('',*,*,#13521,.F.);
#17792=ORIENTED_EDGE('',*,*,#13504,.T.);
#17793=ORIENTED_EDGE('',*,*,#13519,.F.);
#17794=ORIENTED_EDGE('',*,*,#13530,.F.);
#17795=ORIENTED_EDGE('',*,*,#13545,.F.);
#17796=ORIENTED_EDGE('',*,*,#13461,.T.);
#17797=ORIENTED_EDGE('',*,*,#13512,.F.);
#17798=ORIENTED_EDGE('',*,*,#13532,.F.);
#17799=ORIENTED_EDGE('',*,*,#13632,.T.);
#17800=ORIENTED_EDGE('',*,*,#13429,.F.);
#17801=ORIENTED_EDGE('',*,*,#13402,.F.);
#17802=ORIENTED_EDGE('',*,*,#13430,.F.);
#17803=ORIENTED_EDGE('',*,*,#13632,.F.);
#17804=ORIENTED_EDGE('',*,*,#13531,.F.);
#17805=ORIENTED_EDGE('',*,*,#13612,.F.);
#17806=ORIENTED_EDGE('',*,*,#13633,.T.);
#17807=ORIENTED_EDGE('',*,*,#13369,.F.);
#17808=ORIENTED_EDGE('',*,*,#13633,.F.);
#17809=ORIENTED_EDGE('',*,*,#13634,.T.);
#17810=ORIENTED_EDGE('',*,*,#13375,.T.);
#17811=ORIENTED_EDGE('',*,*,#13634,.F.);
#17812=ORIENTED_EDGE('',*,*,#13635,.T.);
#17813=ORIENTED_EDGE('',*,*,#13379,.T.);
#17814=ORIENTED_EDGE('',*,*,#13635,.F.);
#17815=ORIENTED_EDGE('',*,*,#13636,.T.);
#17816=ORIENTED_EDGE('',*,*,#13383,.T.);
#17817=ORIENTED_EDGE('',*,*,#13636,.F.);
#17818=ORIENTED_EDGE('',*,*,#13637,.T.);
#17819=ORIENTED_EDGE('',*,*,#13387,.T.);
#17820=ORIENTED_EDGE('',*,*,#13637,.F.);
#17821=ORIENTED_EDGE('',*,*,#13395,.F.);
#17822=ORIENTED_EDGE('',*,*,#13638,.T.);
#17823=ORIENTED_EDGE('',*,*,#13639,.T.);
#17824=ORIENTED_EDGE('',*,*,#13400,.F.);
#17825=ORIENTED_EDGE('',*,*,#13390,.F.);
#17826=ORIENTED_EDGE('',*,*,#13399,.T.);
#17827=ORIENTED_EDGE('',*,*,#13640,.T.);
#17828=ORIENTED_EDGE('',*,*,#13638,.F.);
#17829=ORIENTED_EDGE('',*,*,#13398,.F.);
#17830=ORIENTED_EDGE('',*,*,#13401,.F.);
#17831=ORIENTED_EDGE('',*,*,#13639,.F.);
#17832=ORIENTED_EDGE('',*,*,#13640,.F.);
#17833=ORIENTED_EDGE('',*,*,#13523,.F.);
#17834=ORIENTED_EDGE('',*,*,#13459,.F.);
#17835=ORIENTED_EDGE('',*,*,#13597,.F.);
#17836=ORIENTED_EDGE('',*,*,#13541,.T.);
#24925=CONICAL_SURFACE('',#26907,1.15732233047034,1.17809724509618);
#24926=CONICAL_SURFACE('',#26911,1.15732233047033,1.17809724509616);
#24927=CONICAL_SURFACE('',#26915,1.15732233047033,1.17809724509616);
#24928=CONICAL_SURFACE('',#26919,1.15732233047034,1.17809724509617);
#24929=CONICAL_SURFACE('',#26924,1.075,0.785398163397438);
#24930=CONICAL_SURFACE('',#26927,1.07500000000001,0.785398163397438);
#24931=CONICAL_SURFACE('',#26934,0.530000000000003,0.785398163397457);
#24932=CONICAL_SURFACE('',#26948,0.530000000000003,0.785398163397457);
#24933=CONICAL_SURFACE('',#26952,0.529999999999999,0.785398163397457);
#24934=CONICAL_SURFACE('',#26956,0.529999999999999,0.785398163397457);
#24935=CONICAL_SURFACE('',#26968,1.01767766952966,0.392699081698724);
#24936=CONICAL_SURFACE('',#26972,1.01767766952966,0.392699081698724);
#24937=CONICAL_SURFACE('',#26977,1.01767766952967,0.392699081698667);
#24938=CONICAL_SURFACE('',#26980,1.01767766952966,0.392699081698703);
#24939=CONICAL_SURFACE('',#27007,1.84267766952967,1.17809724509616);
#24940=CONICAL_SURFACE('',#27010,1.84267766952967,1.17809724509616);
#24941=CONICAL_SURFACE('',#27013,1.84267766952966,1.17809724509616);
#24942=CONICAL_SURFACE('',#27016,1.84267766952966,1.17809724509618);
#24943=CONICAL_SURFACE('',#27020,1.925,0.785398163397446);
#24944=CONICAL_SURFACE('',#27023,1.925,0.785398163397438);
#24945=CONICAL_SURFACE('',#27026,1.98232233047034,0.392699081698708);
#24946=CONICAL_SURFACE('',#27031,1.98232233047034,0.392699081698714);
#24947=CONICAL_SURFACE('',#27035,1.98232233047034,0.392699081698739);
#24948=CONICAL_SURFACE('',#27038,1.98232233047034,0.392699081698699);
#24949=CONICAL_SURFACE('',#27049,1.98232233047034,0.392699081698715);
#24950=CONICAL_SURFACE('',#27053,1.98232233047033,0.392699081698728);
#24951=CONICAL_SURFACE('',#27056,1.95,0.78539816339746);
#24952=CONICAL_SURFACE('',#27059,1.95,0.785398163397448);
#24953=CONICAL_SURFACE('',#27064,1.89267766952966,1.17809724509616);
#24954=CONICAL_SURFACE('',#27068,1.89267766952966,1.17809724509617);
#24955=CONICAL_SURFACE('',#27078,1.98232233047033,0.392699081698725);
#24956=CONICAL_SURFACE('',#27081,1.98232233047034,0.392699081698759);
#24957=CONICAL_SURFACE('',#27089,1.95,0.78539816339746);
#24958=CONICAL_SURFACE('',#27092,1.95,0.785398163397448);
#24959=CONICAL_SURFACE('',#27122,1.075,0.785398163397446);
#24960=CONICAL_SURFACE('',#27124,1.075,0.785398163397446);
#24961=CONICAL_SURFACE('',#27126,1.925,0.785398163397446);
#24962=CONICAL_SURFACE('',#27128,1.925,0.785398163397438);
#24963=CONICAL_SURFACE('',#27133,0.252500000000001,1.02974425867666);
#24964=CONICAL_SURFACE('',#27134,0.252500000000001,1.02974425867666);
#24965=CONICAL_SURFACE('',#27135,0.2525,1.02974425867665);
#24966=CONICAL_SURFACE('',#27136,0.2525,1.02974425867665);
#25112=ADVANCED_FACE('',(#2524),#24925,.F.);
#25113=ADVANCED_FACE('',(#2525),#1656,.T.);
#25114=ADVANCED_FACE('',(#2526),#24926,.F.);
#25115=ADVANCED_FACE('',(#2527),#1657,.T.);
#25116=ADVANCED_FACE('',(#2528),#24927,.F.);
#25117=ADVANCED_FACE('',(#2529),#1658,.T.);
#25118=ADVANCED_FACE('',(#2530),#24928,.F.);
#25119=ADVANCED_FACE('',(#2531),#1659,.T.);
#25120=ADVANCED_FACE('',(#2532),#1660,.T.);
#25121=ADVANCED_FACE('',(#2533),#24929,.F.);
#25122=ADVANCED_FACE('',(#2534),#1661,.T.);
#25123=ADVANCED_FACE('',(#2535),#24930,.F.);
#25124=ADVANCED_FACE('',(#2536,#1553),#1662,.T.);
#25125=ADVANCED_FACE('',(#2537),#24931,.F.);
#25126=ADVANCED_FACE('',(#2538,#1554,#1555,#1556,#1557,#1558,#1559),#1663,
 .T.);
#25127=ADVANCED_FACE('',(#2539),#1103,.F.);
#25128=ADVANCED_FACE('',(#2540),#24932,.F.);
#25129=ADVANCED_FACE('',(#2541),#1104,.F.);
#25130=ADVANCED_FACE('',(#2542),#24933,.F.);
#25131=ADVANCED_FACE('',(#2543),#1105,.F.);
#25132=ADVANCED_FACE('',(#2544),#24934,.F.);
#25133=ADVANCED_FACE('',(#2545),#1106,.F.);
#25134=ADVANCED_FACE('',(#2546),#1664,.T.);
#25135=ADVANCED_FACE('',(#2547),#1665,.T.);
#25136=ADVANCED_FACE('',(#2548),#1666,.T.);
#25137=ADVANCED_FACE('',(#2549),#1667,.T.);
#25138=ADVANCED_FACE('',(#2550),#1668,.F.);
#25139=ADVANCED_FACE('',(#2551),#1669,.F.);
#25140=ADVANCED_FACE('',(#2552),#1670,.T.);
#25141=ADVANCED_FACE('',(#2553),#24935,.F.);
#25142=ADVANCED_FACE('',(#2554),#1671,.T.);
#25143=ADVANCED_FACE('',(#2555),#24936,.F.);
#25144=ADVANCED_FACE('',(#2556),#1672,.T.);
#25145=ADVANCED_FACE('',(#2557),#24937,.F.);
#25146=ADVANCED_FACE('',(#2558),#1673,.T.);
#25147=ADVANCED_FACE('',(#2559),#24938,.F.);
#25148=ADVANCED_FACE('',(#2560),#1674,.F.);
#25149=ADVANCED_FACE('',(#2561),#1107,.F.);
#25150=ADVANCED_FACE('',(#2562),#1675,.F.);
#25151=ADVANCED_FACE('',(#2563),#1108,.F.);
#25152=ADVANCED_FACE('',(#2564),#1676,.F.);
#25153=ADVANCED_FACE('',(#2565),#1109,.F.);
#25154=ADVANCED_FACE('',(#2566),#1677,.T.);
#25155=ADVANCED_FACE('',(#2567),#1678,.T.);
#25156=ADVANCED_FACE('',(#2568),#1679,.T.);
#25157=ADVANCED_FACE('',(#2569),#1680,.T.);
#25158=ADVANCED_FACE('',(#2570),#1681,.T.);
#25159=ADVANCED_FACE('',(#2571),#1682,.T.);
#25160=ADVANCED_FACE('',(#2572),#1683,.T.);
#25161=ADVANCED_FACE('',(#2573),#1684,.T.);
#25162=ADVANCED_FACE('',(#2574),#1685,.T.);
#25163=ADVANCED_FACE('',(#2575),#1686,.T.);
#25164=ADVANCED_FACE('',(#2576),#24939,.T.);
#25165=ADVANCED_FACE('',(#2577),#1687,.T.);
#25166=ADVANCED_FACE('',(#2578),#24940,.T.);
#25167=ADVANCED_FACE('',(#2579),#1688,.T.);
#25168=ADVANCED_FACE('',(#2580),#24941,.T.);
#25169=ADVANCED_FACE('',(#2581),#1689,.T.);
#25170=ADVANCED_FACE('',(#2582),#24942,.T.);
#25171=ADVANCED_FACE('',(#2583),#1690,.T.);
#25172=ADVANCED_FACE('',(#2584),#1691,.T.);
#25173=ADVANCED_FACE('',(#2585),#24943,.T.);
#25174=ADVANCED_FACE('',(#2586),#1692,.T.);
#25175=ADVANCED_FACE('',(#2587),#24944,.T.);
#25176=ADVANCED_FACE('',(#2588),#1693,.T.);
#25177=ADVANCED_FACE('',(#2589),#24945,.T.);
#25178=ADVANCED_FACE('',(#2590),#1694,.T.);
#25179=ADVANCED_FACE('',(#2591),#24946,.T.);
#25180=ADVANCED_FACE('',(#2592),#1695,.T.);
#25181=ADVANCED_FACE('',(#2593),#24947,.T.);
#25182=ADVANCED_FACE('',(#2594),#1696,.T.);
#25183=ADVANCED_FACE('',(#2595),#24948,.T.);
#25184=ADVANCED_FACE('',(#2596),#1697,.T.);
#25185=ADVANCED_FACE('',(#2597),#1110,.T.);
#25186=ADVANCED_FACE('',(#2598),#1698,.T.);
#25187=ADVANCED_FACE('',(#2599),#1111,.T.);
#25188=ADVANCED_FACE('',(#2600),#1699,.T.);
#25189=ADVANCED_FACE('',(#2601),#24949,.T.);
#25190=ADVANCED_FACE('',(#2602),#1700,.T.);
#25191=ADVANCED_FACE('',(#2603),#24950,.T.);
#25192=ADVANCED_FACE('',(#2604),#1701,.T.);
#25193=ADVANCED_FACE('',(#2605),#24951,.T.);
#25194=ADVANCED_FACE('',(#2606),#1702,.T.);
#25195=ADVANCED_FACE('',(#2607),#24952,.T.);
#25196=ADVANCED_FACE('',(#2608),#1703,.T.);
#25197=ADVANCED_FACE('',(#2609),#1704,.T.);
#25198=ADVANCED_FACE('',(#2610),#1705,.T.);
#25199=ADVANCED_FACE('',(#2611),#24953,.T.);
#25200=ADVANCED_FACE('',(#2612),#1706,.T.);
#25201=ADVANCED_FACE('',(#2613),#24954,.T.);
#25202=ADVANCED_FACE('',(#2614),#1707,.T.);
#25203=ADVANCED_FACE('',(#2615),#1708,.T.);
#25204=ADVANCED_FACE('',(#2616),#1709,.T.);
#25205=ADVANCED_FACE('',(#2617),#1710,.T.);
#25206=ADVANCED_FACE('',(#2618),#1711,.T.);
#25207=ADVANCED_FACE('',(#2619),#1712,.T.);
#25208=ADVANCED_FACE('',(#2620),#1713,.T.);
#25209=ADVANCED_FACE('',(#2621),#24955,.T.);
#25210=ADVANCED_FACE('',(#2622),#1714,.T.);
#25211=ADVANCED_FACE('',(#2623),#24956,.T.);
#25212=ADVANCED_FACE('',(#2624),#1715,.T.);
#25213=ADVANCED_FACE('',(#2625),#1716,.T.);
#25214=ADVANCED_FACE('',(#2626),#1717,.T.);
#25215=ADVANCED_FACE('',(#2627),#1718,.T.);
#25216=ADVANCED_FACE('',(#2628),#1719,.T.);
#25217=ADVANCED_FACE('',(#2629),#24957,.T.);
#25218=ADVANCED_FACE('',(#2630),#1720,.T.);
#25219=ADVANCED_FACE('',(#2631),#1721,.T.);
#25220=ADVANCED_FACE('',(#2632),#24958,.T.);
#25221=ADVANCED_FACE('',(#2633),#1722,.F.);
#25222=ADVANCED_FACE('',(#2634,#1560),#1723,.F.);
#25223=ADVANCED_FACE('',(#2635),#1724,.F.);
#25224=ADVANCED_FACE('',(#2636),#1725,.F.);
#25225=ADVANCED_FACE('',(#2637),#1726,.T.);
#25226=ADVANCED_FACE('',(#2638),#1727,.T.);
#25227=ADVANCED_FACE('',(#2639),#1728,.F.);
#25228=ADVANCED_FACE('',(#2640),#1079,.F.);
#25229=ADVANCED_FACE('',(#2641),#1112,.F.);
#25230=ADVANCED_FACE('',(#2642),#1080,.F.);
#25231=ADVANCED_FACE('',(#2643),#1113,.F.);
#25232=ADVANCED_FACE('',(#2644),#1081,.F.);
#25233=ADVANCED_FACE('',(#2645),#1114,.F.);
#25234=ADVANCED_FACE('',(#2646),#1082,.F.);
#25235=ADVANCED_FACE('',(#2647),#1115,.F.);
#25236=ADVANCED_FACE('',(#2648),#1116,.F.);
#25237=ADVANCED_FACE('',(#2649),#1729,.F.);
#25238=ADVANCED_FACE('',(#2650),#1117,.F.);
#25239=ADVANCED_FACE('',(#2651),#24959,.F.);
#25240=ADVANCED_FACE('',(#2652),#1730,.T.);
#25241=ADVANCED_FACE('',(#2653),#24960,.F.);
#25242=ADVANCED_FACE('',(#2654),#1731,.T.);
#25243=ADVANCED_FACE('',(#2655),#24961,.T.);
#25244=ADVANCED_FACE('',(#2656),#1732,.T.);
#25245=ADVANCED_FACE('',(#2657),#24962,.T.);
#25246=ADVANCED_FACE('',(#2658),#1733,.T.);
#25247=ADVANCED_FACE('',(#2659),#1118,.T.);
#25248=ADVANCED_FACE('',(#2660),#1119,.F.);
#25249=ADVANCED_FACE('',(#2661),#1120,.F.);
#25250=ADVANCED_FACE('',(#2662),#24963,.F.);
#25251=ADVANCED_FACE('',(#2663),#24964,.F.);
#25252=ADVANCED_FACE('',(#2664),#24965,.F.);
#25253=ADVANCED_FACE('',(#2665),#24966,.F.);
#25254=ADVANCED_FACE('',(#2666),#1734,.F.);
#25255=ADVANCED_FACE('',(#2667),#1735,.F.);
#25256=ADVANCED_FACE('',(#2668),#1736,.F.);
#25257=ADVANCED_FACE('',(#2669),#1121,.T.);
#26664=CLOSED_SHELL('',(#25112,#25113,#25114,#25115,#25116,#25117,#25118,
#25119,#25120,#25121,#25122,#25123,#25124,#25125,#25126,#25127,#25128,#25129,
#25130,#25131,#25132,#25133,#25134,#25135,#25136,#25137,#25138,#25139,#25140,
#25141,#25142,#25143,#25144,#25145,#25146,#25147,#25148,#25149,#25150,#25151,
#25152,#25153,#25154,#25155,#25156,#25157,#25158,#25159,#25160,#25161,#25162,
#25163,#25164,#25165,#25166,#25167,#25168,#25169,#25170,#25171,#25172,#25173,
#25174,#25175,#25176,#25177,#25178,#25179,#25180,#25181,#25182,#25183,#25184,
#25185,#25186,#25187,#25188,#25189,#25190,#25191,#25192,#25193,#25194,#25195,
#25196,#25197,#25198,#25199,#25200,#25201,#25202,#25203,#25204,#25205,#25206,
#25207,#25208,#25209,#25210,#25211,#25212,#25213,#25214,#25215,#25216,#25217,
#25218,#25219,#25220,#25221,#25222,#25223,#25224,#25225,#25226,#25227,#25228,
#25229,#25230,#25231,#25232,#25233,#25234,#25235,#25236,#25237,#25238,#25239,
#25240,#25241,#25242,#25243,#25244,#25245,#25246,#25247,#25248,#25249,#25250,
#25251,#25252,#25253,#25254,#25255,#25256,#25257));
#26906=AXIS2_PLACEMENT_3D('',#36382,#29347,#29348);
#26907=AXIS2_PLACEMENT_3D('',#36383,#29349,#29350);
#26908=AXIS2_PLACEMENT_3D('',#36388,#29352,#29353);
#26909=AXIS2_PLACEMENT_3D('',#36391,#29355,#29356);
#26910=AXIS2_PLACEMENT_3D('',#36392,#29357,#29358);
#26911=AXIS2_PLACEMENT_3D('',#36398,#29362,#29363);
#26912=AXIS2_PLACEMENT_3D('',#36402,#29365,#29366);
#26913=AXIS2_PLACEMENT_3D('',#36403,#29367,#29368);
#26914=AXIS2_PLACEMENT_3D('',#36404,#29369,#29370);
#26915=AXIS2_PLACEMENT_3D('',#36410,#29374,#29375);
#26916=AXIS2_PLACEMENT_3D('',#36414,#29377,#29378);
#26917=AXIS2_PLACEMENT_3D('',#36415,#29379,#29380);
#26918=AXIS2_PLACEMENT_3D('',#36416,#29381,#29382);
#26919=AXIS2_PLACEMENT_3D('',#36422,#29386,#29387);
#26920=AXIS2_PLACEMENT_3D('',#36426,#29389,#29390);
#26921=AXIS2_PLACEMENT_3D('',#36427,#29391,#29392);
#26922=AXIS2_PLACEMENT_3D('',#36428,#29393,#29394);
#26923=AXIS2_PLACEMENT_3D('',#36431,#29397,#29398);
#26924=AXIS2_PLACEMENT_3D('',#36437,#29402,#29403);
#26925=AXIS2_PLACEMENT_3D('',#36440,#29405,#29406);
#26926=AXIS2_PLACEMENT_3D('',#36441,#29407,#29408);
#26927=AXIS2_PLACEMENT_3D('',#36445,#29411,#29412);
#26928=AXIS2_PLACEMENT_3D('',#36448,#29414,#29415);
#26929=AXIS2_PLACEMENT_3D('',#36449,#29416,#29417);
#26930=AXIS2_PLACEMENT_3D('',#36452,#29418,#29419);
#26931=AXIS2_PLACEMENT_3D('',#36456,#29421,#29422);
#26932=AXIS2_PLACEMENT_3D('',#36460,#29424,#29425);
#26933=AXIS2_PLACEMENT_3D('',#36464,#29427,#29428);
#26934=AXIS2_PLACEMENT_3D('',#36466,#29430,#29431);
#26935=AXIS2_PLACEMENT_3D('',#36468,#29432,#29433);
#26936=AXIS2_PLACEMENT_3D('',#36471,#29435,#29436);
#26937=AXIS2_PLACEMENT_3D('',#36472,#29437,#29438);
#26938=AXIS2_PLACEMENT_3D('',#36475,#29439,#29440);
#26939=AXIS2_PLACEMENT_3D('',#36479,#29442,#29443);
#26940=AXIS2_PLACEMENT_3D('',#36483,#29445,#29446);
#26941=AXIS2_PLACEMENT_3D('',#36487,#29448,#29449);
#26942=AXIS2_PLACEMENT_3D('',#36490,#29451,#29452);
#26943=AXIS2_PLACEMENT_3D('',#36492,#29453,#29454);
#26944=AXIS2_PLACEMENT_3D('',#36494,#29455,#29456);
#26945=AXIS2_PLACEMENT_3D('',#36504,#29461,#29462);
#26946=AXIS2_PLACEMENT_3D('',#36505,#29463,#29464);
#26947=AXIS2_PLACEMENT_3D('',#36507,#29465,#29466);
#26948=AXIS2_PLACEMENT_3D('',#36509,#29468,#29469);
#26949=AXIS2_PLACEMENT_3D('',#36512,#29471,#29472);
#26950=AXIS2_PLACEMENT_3D('',#36513,#29473,#29474);
#26951=AXIS2_PLACEMENT_3D('',#36515,#29475,#29476);
#26952=AXIS2_PLACEMENT_3D('',#36517,#29478,#29479);
#26953=AXIS2_PLACEMENT_3D('',#36520,#29481,#29482);
#26954=AXIS2_PLACEMENT_3D('',#36521,#29483,#29484);
#26955=AXIS2_PLACEMENT_3D('',#36523,#29485,#29486);
#26956=AXIS2_PLACEMENT_3D('',#36525,#29488,#29489);
#26957=AXIS2_PLACEMENT_3D('',#36528,#29491,#29492);
#26958=AXIS2_PLACEMENT_3D('',#36529,#29493,#29494);
#26959=AXIS2_PLACEMENT_3D('',#36531,#29495,#29496);
#26960=AXIS2_PLACEMENT_3D('',#36533,#29498,#29499);
#26961=AXIS2_PLACEMENT_3D('',#36539,#29503,#29504);
#26962=AXIS2_PLACEMENT_3D('',#36545,#29508,#29509);
#26963=AXIS2_PLACEMENT_3D('',#36547,#29511,#29512);
#26964=AXIS2_PLACEMENT_3D('',#36549,#29514,#29515);
#26965=AXIS2_PLACEMENT_3D('',#36555,#29519,#29520);
#26966=AXIS2_PLACEMENT_3D('',#36559,#29523,#29524);
#26967=AXIS2_PLACEMENT_3D('',#36562,#29525,#29526);
#26968=AXIS2_PLACEMENT_3D('',#36569,#29531,#29532);
#26969=AXIS2_PLACEMENT_3D('',#36573,#29534,#29535);
#26970=AXIS2_PLACEMENT_3D('',#36574,#29536,#29537);
#26971=AXIS2_PLACEMENT_3D('',#36575,#29538,#29539);
#26972=AXIS2_PLACEMENT_3D('',#36581,#29543,#29544);
#26973=AXIS2_PLACEMENT_3D('',#36585,#29546,#29547);
#26974=AXIS2_PLACEMENT_3D('',#36586,#29548,#29549);
#26975=AXIS2_PLACEMENT_3D('',#36587,#29550,#29551);
#26976=AXIS2_PLACEMENT_3D('',#36590,#29552,#29553);
#26977=AXIS2_PLACEMENT_3D('',#36596,#29558,#29559);
#26978=AXIS2_PLACEMENT_3D('',#36599,#29561,#29562);
#26979=AXIS2_PLACEMENT_3D('',#36600,#29563,#29564);
#26980=AXIS2_PLACEMENT_3D('',#36604,#29567,#29568);
#26981=AXIS2_PLACEMENT_3D('',#36605,#29569,#29570);
#26982=AXIS2_PLACEMENT_3D('',#36606,#29571,#29572);
#26983=AXIS2_PLACEMENT_3D('',#36613,#29576,#29577);
#26984=AXIS2_PLACEMENT_3D('',#36614,#29578,#29579);
#26985=AXIS2_PLACEMENT_3D('',#36615,#29580,#29581);
#26986=AXIS2_PLACEMENT_3D('',#36618,#29583,#29584);
#26987=AXIS2_PLACEMENT_3D('',#36619,#29585,#29586);
#26988=AXIS2_PLACEMENT_3D('',#36623,#29589,#29590);
#26989=AXIS2_PLACEMENT_3D('',#36626,#29592,#29593);
#26990=AXIS2_PLACEMENT_3D('',#36627,#29594,#29595);
#26991=AXIS2_PLACEMENT_3D('',#36629,#29596,#29597);
#26992=AXIS2_PLACEMENT_3D('',#36630,#29598,#29599);
#26993=AXIS2_PLACEMENT_3D('',#36634,#29602,#29603);
#26994=AXIS2_PLACEMENT_3D('',#36638,#29605,#29606);
#26995=AXIS2_PLACEMENT_3D('',#36640,#29607,#29608);
#26996=AXIS2_PLACEMENT_3D('',#36641,#29609,#29610);
#26997=AXIS2_PLACEMENT_3D('',#36642,#29611,#29612);
#26998=AXIS2_PLACEMENT_3D('',#36653,#29618,#29619);
#26999=AXIS2_PLACEMENT_3D('',#36659,#29623,#29624);
#27000=AXIS2_PLACEMENT_3D('',#36667,#29629,#29630);
#27001=AXIS2_PLACEMENT_3D('',#36677,#29636,#29637);
#27002=AXIS2_PLACEMENT_3D('',#36685,#29642,#29643);
#27003=AXIS2_PLACEMENT_3D('',#36693,#29648,#29649);
#27004=AXIS2_PLACEMENT_3D('',#36699,#29653,#29654);
#27005=AXIS2_PLACEMENT_3D('',#36705,#29658,#29659);
#27006=AXIS2_PLACEMENT_3D('',#36711,#29663,#29664);
#27007=AXIS2_PLACEMENT_3D('',#36715,#29667,#29668);
#27008=AXIS2_PLACEMENT_3D('',#36719,#29670,#29671);
#27009=AXIS2_PLACEMENT_3D('',#36721,#29673,#29674);
#27010=AXIS2_PLACEMENT_3D('',#36725,#29677,#29678);
#27011=AXIS2_PLACEMENT_3D('',#36728,#29680,#29681);
#27012=AXIS2_PLACEMENT_3D('',#36729,#29682,#29683);
#27013=AXIS2_PLACEMENT_3D('',#36733,#29686,#29687);
#27014=AXIS2_PLACEMENT_3D('',#36736,#29689,#29690);
#27015=AXIS2_PLACEMENT_3D('',#36737,#29691,#29692);
#27016=AXIS2_PLACEMENT_3D('',#36741,#29695,#29696);
#27017=AXIS2_PLACEMENT_3D('',#36744,#29698,#29699);
#27018=AXIS2_PLACEMENT_3D('',#36745,#29700,#29701);
#27019=AXIS2_PLACEMENT_3D('',#36747,#29703,#29704);
#27020=AXIS2_PLACEMENT_3D('',#36753,#29708,#29709);
#27021=AXIS2_PLACEMENT_3D('',#36756,#29711,#29712);
#27022=AXIS2_PLACEMENT_3D('',#36757,#29713,#29714);
#27023=AXIS2_PLACEMENT_3D('',#36761,#29717,#29718);
#27024=AXIS2_PLACEMENT_3D('',#36764,#29720,#29721);
#27025=AXIS2_PLACEMENT_3D('',#36765,#29722,#29723);
#27026=AXIS2_PLACEMENT_3D('',#36771,#29727,#29728);
#27027=AXIS2_PLACEMENT_3D('',#36775,#29730,#29731);
#27028=AXIS2_PLACEMENT_3D('',#36776,#29732,#29733);
#27029=AXIS2_PLACEMENT_3D('',#36777,#29734,#29735);
#27030=AXIS2_PLACEMENT_3D('',#36780,#29736,#29737);
#27031=AXIS2_PLACEMENT_3D('',#36787,#29742,#29743);
#27032=AXIS2_PLACEMENT_3D('',#36790,#29745,#29746);
#27033=AXIS2_PLACEMENT_3D('',#36791,#29747,#29748);
#27034=AXIS2_PLACEMENT_3D('',#36792,#29749,#29750);
#27035=AXIS2_PLACEMENT_3D('',#36795,#29753,#29754);
#27036=AXIS2_PLACEMENT_3D('',#36798,#29756,#29757);
#27037=AXIS2_PLACEMENT_3D('',#36799,#29758,#29759);
#27038=AXIS2_PLACEMENT_3D('',#36804,#29763,#29764);
#27039=AXIS2_PLACEMENT_3D('',#36805,#29765,#29766);
#27040=AXIS2_PLACEMENT_3D('',#36806,#29767,#29768);
#27041=AXIS2_PLACEMENT_3D('',#36813,#29772,#29773);
#27042=AXIS2_PLACEMENT_3D('',#36814,#29774,#29775);
#27043=AXIS2_PLACEMENT_3D('',#36815,#29776,#29777);
#27044=AXIS2_PLACEMENT_3D('',#36817,#29779,#29780);
#27045=AXIS2_PLACEMENT_3D('',#36818,#29781,#29782);
#27046=AXIS2_PLACEMENT_3D('',#36826,#29787,#29788);
#27047=AXIS2_PLACEMENT_3D('',#36829,#29790,#29791);
#27048=AXIS2_PLACEMENT_3D('',#36830,#29792,#29793);
#27049=AXIS2_PLACEMENT_3D('',#36834,#29796,#29797);
#27050=AXIS2_PLACEMENT_3D('',#36837,#29799,#29800);
#27051=AXIS2_PLACEMENT_3D('',#36838,#29801,#29802);
#27052=AXIS2_PLACEMENT_3D('',#36839,#29803,#29804);
#27053=AXIS2_PLACEMENT_3D('',#36843,#29807,#29808);
#27054=AXIS2_PLACEMENT_3D('',#36844,#29809,#29810);
#27055=AXIS2_PLACEMENT_3D('',#36845,#29811,#29812);
#27056=AXIS2_PLACEMENT_3D('',#36849,#29815,#29816);
#27057=AXIS2_PLACEMENT_3D('',#36852,#29818,#29819);
#27058=AXIS2_PLACEMENT_3D('',#36853,#29820,#29821);
#27059=AXIS2_PLACEMENT_3D('',#36857,#29824,#29825);
#27060=AXIS2_PLACEMENT_3D('',#36858,#29826,#29827);
#27061=AXIS2_PLACEMENT_3D('',#36859,#29828,#29829);
#27062=AXIS2_PLACEMENT_3D('',#36866,#29833,#29834);
#27063=AXIS2_PLACEMENT_3D('',#36873,#29838,#29839);
#27064=AXIS2_PLACEMENT_3D('',#36879,#29843,#29844);
#27065=AXIS2_PLACEMENT_3D('',#36883,#29846,#29847);
#27066=AXIS2_PLACEMENT_3D('',#36884,#29848,#29849);
#27067=AXIS2_PLACEMENT_3D('',#36885,#29850,#29851);
#27068=AXIS2_PLACEMENT_3D('',#36891,#29855,#29856);
#27069=AXIS2_PLACEMENT_3D('',#36895,#29858,#29859);
#27070=AXIS2_PLACEMENT_3D('',#36896,#29860,#29861);
#27071=AXIS2_PLACEMENT_3D('',#36897,#29862,#29863);
#27072=AXIS2_PLACEMENT_3D('',#36900,#29866,#29867);
#27073=AXIS2_PLACEMENT_3D('',#36903,#29870,#29871);
#27074=AXIS2_PLACEMENT_3D('',#36911,#29876,#29877);
#27075=AXIS2_PLACEMENT_3D('',#36919,#29882,#29883);
#27076=AXIS2_PLACEMENT_3D('',#36923,#29886,#29887);
#27077=AXIS2_PLACEMENT_3D('',#36925,#29889,#29890);
#27078=AXIS2_PLACEMENT_3D('',#36929,#29893,#29894);
#27079=AXIS2_PLACEMENT_3D('',#36932,#29896,#29897);
#27080=AXIS2_PLACEMENT_3D('',#36933,#29898,#29899);
#27081=AXIS2_PLACEMENT_3D('',#36937,#29902,#29903);
#27082=AXIS2_PLACEMENT_3D('',#36940,#29905,#29906);
#27083=AXIS2_PLACEMENT_3D('',#36941,#29907,#29908);
#27084=AXIS2_PLACEMENT_3D('',#36942,#29909,#29910);
#27085=AXIS2_PLACEMENT_3D('',#36944,#29912,#29913);
#27086=AXIS2_PLACEMENT_3D('',#36947,#29916,#29917);
#27087=AXIS2_PLACEMENT_3D('',#36950,#29920,#29921);
#27088=AXIS2_PLACEMENT_3D('',#36952,#29923,#29924);
#27089=AXIS2_PLACEMENT_3D('',#36955,#29927,#29928);
#27090=AXIS2_PLACEMENT_3D('',#36958,#29931,#29932);
#27091=AXIS2_PLACEMENT_3D('',#36960,#29934,#29935);
#27092=AXIS2_PLACEMENT_3D('',#36962,#29937,#29938);
#27093=AXIS2_PLACEMENT_3D('',#36963,#29939,#29940);
#27094=AXIS2_PLACEMENT_3D('',#36965,#29942,#29943);
#27095=AXIS2_PLACEMENT_3D('',#36968,#29945,#29946);
#27096=AXIS2_PLACEMENT_3D('',#36969,#29947,#29948);
#27097=AXIS2_PLACEMENT_3D('',#36970,#29949,#29950);
#27098=AXIS2_PLACEMENT_3D('',#36971,#29951,#29952);
#27099=AXIS2_PLACEMENT_3D('',#36972,#29953,#29954);
#27100=AXIS2_PLACEMENT_3D('',#36973,#29955,#29956);
#27101=AXIS2_PLACEMENT_3D('',#36974,#29957,#29958);
#27102=AXIS2_PLACEMENT_3D('',#36976,#29959,#29960);
#27103=AXIS2_PLACEMENT_3D('',#36977,#29961,#29962);
#27104=AXIS2_PLACEMENT_3D('',#36978,#29963,#29964);
#27105=AXIS2_PLACEMENT_3D('',#36979,#29965,#29966);
#27106=AXIS2_PLACEMENT_3D('',#36980,#29967,#29968);
#27107=AXIS2_PLACEMENT_3D('',#36981,#29969,#29970);
#27108=AXIS2_PLACEMENT_3D('',#36982,#29971,#29972);
#27109=AXIS2_PLACEMENT_3D('',#36983,#29973,#29974);
#27110=AXIS2_PLACEMENT_3D('',#36984,#29975,#29976);
#27111=AXIS2_PLACEMENT_3D('',#36985,#29977,#29978);
#27112=AXIS2_PLACEMENT_3D('',#36986,#29979,#29980);
#27113=AXIS2_PLACEMENT_3D('',#36987,#29981,#29982);
#27114=AXIS2_PLACEMENT_3D('',#36988,#29983,#29984);
#27115=AXIS2_PLACEMENT_3D('',#36989,#29985,#29986);
#27116=AXIS2_PLACEMENT_3D('',#36991,#29987,#29988);
#27117=AXIS2_PLACEMENT_3D('',#36992,#29989,#29990);
#27118=AXIS2_PLACEMENT_3D('',#36993,#29991,#29992);
#27119=AXIS2_PLACEMENT_3D('',#36995,#29994,#29995);
#27120=AXIS2_PLACEMENT_3D('',#36997,#29997,#29998);
#27121=AXIS2_PLACEMENT_3D('',#36999,#30000,#30001);
#27122=AXIS2_PLACEMENT_3D('',#37000,#30002,#30003);
#27123=AXIS2_PLACEMENT_3D('',#37002,#30005,#30006);
#27124=AXIS2_PLACEMENT_3D('',#37004,#30008,#30009);
#27125=AXIS2_PLACEMENT_3D('',#37006,#30011,#30012);
#27126=AXIS2_PLACEMENT_3D('',#37007,#30013,#30014);
#27127=AXIS2_PLACEMENT_3D('',#37009,#30016,#30017);
#27128=AXIS2_PLACEMENT_3D('',#37011,#30019,#30020);
#27129=AXIS2_PLACEMENT_3D('',#37013,#30022,#30023);
#27130=AXIS2_PLACEMENT_3D('',#37014,#30024,#30025);
#27131=AXIS2_PLACEMENT_3D('',#37015,#30026,#30027);
#27132=AXIS2_PLACEMENT_3D('',#37017,#30029,#30030);
#27133=AXIS2_PLACEMENT_3D('',#37019,#30032,#30033);
#27134=AXIS2_PLACEMENT_3D('',#37022,#30035,#30036);
#27135=AXIS2_PLACEMENT_3D('',#37025,#30038,#30039);
#27136=AXIS2_PLACEMENT_3D('',#37028,#30041,#30042);
#27137=AXIS2_PLACEMENT_3D('',#37031,#30044,#30045);
#27138=AXIS2_PLACEMENT_3D('',#37035,#30048,#30049);
#27139=AXIS2_PLACEMENT_3D('',#37037,#30051,#30052);
#27140=AXIS2_PLACEMENT_3D('',#37038,#30053,#30054);
#29347=DIRECTION('axis',(0.,0.,1.));
#29348=DIRECTION('refdir',(1.,0.,0.));
#29349=DIRECTION('center_axis',(0.,0.,1.));
#29350=DIRECTION('ref_axis',(1.,1.68837364655892E-15,0.));
#29351=DIRECTION('',(0.,-0.923879532511291,-0.38268343236508));
#29352=DIRECTION('center_axis',(1.26986498732449E-30,-7.96826514156151E-16,
-1.));
#29353=DIRECTION('ref_axis',(1.,1.5936530283123E-15,0.));
#29354=DIRECTION('',(0.923879532511289,0.,0.382683432365085));
#29355=DIRECTION('center_axis',(0.,0.,1.));
#29356=DIRECTION('ref_axis',(1.,1.77635683940024E-15,0.));
#29357=DIRECTION('center_axis',(0.,-0.382683432365063,0.923879532511298));
#29358=DIRECTION('ref_axis',(1.,0.,0.));
#29359=DIRECTION('',(0.,-0.923879532511294,-0.382683432365072));
#29360=DIRECTION('',(1.,0.,0.));
#29361=DIRECTION('',(-1.,0.,0.));
#29362=DIRECTION('center_axis',(0.,0.,1.));
#29363=DIRECTION('ref_axis',(1.68837364655893E-15,1.,0.));
#29364=DIRECTION('',(0.923879532511285,0.,-0.382683432365095));
#29365=DIRECTION('center_axis',(0.,0.,-1.));
#29366=DIRECTION('ref_axis',(1.59365302831231E-15,1.,0.));
#29367=DIRECTION('center_axis',(0.,0.,1.));
#29368=DIRECTION('ref_axis',(1.77635683940025E-15,1.,0.));
#29369=DIRECTION('center_axis',(0.382683432365072,0.,0.923879532511294));
#29370=DIRECTION('ref_axis',(0.923879532511294,0.,-0.382683432365072));
#29371=DIRECTION('',(0.923879532511298,0.,-0.382683432365063));
#29372=DIRECTION('',(0.,1.,0.));
#29373=DIRECTION('',(0.,-1.,0.));
#29374=DIRECTION('center_axis',(0.,0.,1.));
#29375=DIRECTION('ref_axis',(-1.,0.,0.));
#29376=DIRECTION('',(0.,0.923879532511282,-0.382683432365102));
#29377=DIRECTION('center_axis',(0.,0.,-1.));
#29378=DIRECTION('ref_axis',(-1.,0.,0.));
#29379=DIRECTION('center_axis',(0.,0.,1.));
#29380=DIRECTION('ref_axis',(-1.,0.,0.));
#29381=DIRECTION('center_axis',(0.,0.382683432365063,0.923879532511298));
#29382=DIRECTION('ref_axis',(1.,0.,0.));
#29383=DIRECTION('',(0.,0.923879532511291,-0.382683432365078));
#29384=DIRECTION('',(-1.,0.,0.));
#29385=DIRECTION('',(1.,0.,0.));
#29386=DIRECTION('center_axis',(0.,0.,1.));
#29387=DIRECTION('ref_axis',(6.75349458623569E-15,-1.,0.));
#29388=DIRECTION('',(-0.923879532511281,-1.92271478790305E-14,-0.382683432365104));
#29389=DIRECTION('center_axis',(1.5936530283123E-15,1.01589198985959E-29,
-1.));
#29390=DIRECTION('ref_axis',(6.37461211324924E-15,-1.,0.));
#29391=DIRECTION('center_axis',(0.,0.,1.));
#29392=DIRECTION('ref_axis',(7.10542735760099E-15,-1.,0.));
#29393=DIRECTION('center_axis',(-0.382683432365085,0.,0.923879532511289));
#29394=DIRECTION('ref_axis',(0.923879532511289,0.,0.382683432365085));
#29395=DIRECTION('',(0.,-1.,0.));
#29396=DIRECTION('',(0.,1.,0.));
#29397=DIRECTION('center_axis',(0.,0.707106781186548,0.707106781186548));
#29398=DIRECTION('ref_axis',(1.,0.,0.));
#29399=DIRECTION('',(0.,0.707106781186548,-0.707106781186548));
#29400=DIRECTION('',(1.,0.,0.));
#29401=DIRECTION('',(8.3738264463134E-15,-0.707106781186552,0.707106781186543));
#29402=DIRECTION('center_axis',(0.,0.,1.));
#29403=DIRECTION('ref_axis',(7.10542735760099E-15,-1.,0.));
#29404=DIRECTION('',(0.707106781186543,0.,0.707106781186552));
#29405=DIRECTION('center_axis',(-1.71569776325697E-15,-1.17744752593799E-29,
1.));
#29406=DIRECTION('ref_axis',(6.86279105302788E-15,-1.,0.));
#29407=DIRECTION('center_axis',(-0.707106781186552,0.,0.707106781186543));
#29408=DIRECTION('ref_axis',(0.707106781186543,0.,0.707106781186552));
#29409=DIRECTION('',(0.707106781186543,0.,0.707106781186552));
#29410=DIRECTION('',(0.,1.,0.));
#29411=DIRECTION('center_axis',(0.,0.,1.));
#29412=DIRECTION('ref_axis',(1.,1.77635683940024E-15,0.));
#29413=DIRECTION('',(0.,0.707106781186548,0.707106781186548));
#29414=DIRECTION('center_axis',(2.94361881484495E-30,-1.71569776325696E-15,
1.));
#29415=DIRECTION('ref_axis',(1.,1.71569776325697E-15,0.));
#29416=DIRECTION('center_axis',(0.,0.,1.));
#29417=DIRECTION('ref_axis',(1.,0.,0.));
#29418=DIRECTION('center_axis',(0.,0.,-1.));
#29419=DIRECTION('ref_axis',(1.,1.77635683940025E-15,0.));
#29420=DIRECTION('',(1.,0.,0.));
#29421=DIRECTION('center_axis',(0.,0.,-1.));
#29422=DIRECTION('ref_axis',(8.88178419700126E-16,1.,0.));
#29423=DIRECTION('',(0.,1.,0.));
#29424=DIRECTION('center_axis',(0.,0.,-1.));
#29425=DIRECTION('ref_axis',(-1.,0.,0.));
#29426=DIRECTION('',(-1.,0.,0.));
#29427=DIRECTION('center_axis',(0.,0.,-1.));
#29428=DIRECTION('ref_axis',(0.,-1.,0.));
#29429=DIRECTION('',(0.,-1.,0.));
#29430=DIRECTION('center_axis',(0.,0.,1.));
#29431=DIRECTION('ref_axis',(1.,0.,0.));
#29432=DIRECTION('center_axis',(0.,0.,1.));
#29433=DIRECTION('ref_axis',(1.,0.,0.));
#29434=DIRECTION('',(0.707106781186554,8.65956056235501E-17,-0.707106781186541));
#29435=DIRECTION('center_axis',(0.,0.,-1.));
#29436=DIRECTION('ref_axis',(1.,0.,0.));
#29437=DIRECTION('center_axis',(0.,0.,1.));
#29438=DIRECTION('ref_axis',(1.,0.,0.));
#29439=DIRECTION('center_axis',(0.,0.,-1.));
#29440=DIRECTION('ref_axis',(-0.707106781186547,0.707106781186548,0.));
#29441=DIRECTION('',(0.,1.,0.));
#29442=DIRECTION('center_axis',(0.,0.,-1.));
#29443=DIRECTION('ref_axis',(-0.707106781186548,-0.707106781186548,0.));
#29444=DIRECTION('',(-1.,0.,0.));
#29445=DIRECTION('center_axis',(0.,0.,-1.));
#29446=DIRECTION('ref_axis',(0.707106781186551,-0.707106781186544,0.));
#29447=DIRECTION('',(0.,-1.,0.));
#29448=DIRECTION('center_axis',(0.,0.,-1.));
#29449=DIRECTION('ref_axis',(0.707106781186548,0.707106781186547,0.));
#29450=DIRECTION('',(1.,0.,0.));
#29451=DIRECTION('center_axis',(0.,0.,1.));
#29452=DIRECTION('ref_axis',(1.,0.,0.));
#29453=DIRECTION('center_axis',(0.,0.,1.));
#29454=DIRECTION('ref_axis',(1.,0.,0.));
#29455=DIRECTION('center_axis',(0.,0.,-1.));
#29456=DIRECTION('ref_axis',(1.,0.,0.));
#29457=DIRECTION('',(1.,0.,0.));
#29458=DIRECTION('',(0.,-1.,0.));
#29459=DIRECTION('',(-1.,0.,0.));
#29460=DIRECTION('',(0.,1.,0.));
#29461=DIRECTION('center_axis',(0.,0.,1.));
#29462=DIRECTION('ref_axis',(1.,0.,0.));
#29463=DIRECTION('center_axis',(0.,0.,1.));
#29464=DIRECTION('ref_axis',(1.,0.,0.));
#29465=DIRECTION('center_axis',(0.,0.,1.));
#29466=DIRECTION('ref_axis',(1.,0.,0.));
#29467=DIRECTION('',(0.,0.,1.));
#29468=DIRECTION('center_axis',(0.,0.,1.));
#29469=DIRECTION('ref_axis',(1.,0.,0.));
#29470=DIRECTION('',(0.707106781186554,8.65956056235501E-17,-0.707106781186541));
#29471=DIRECTION('center_axis',(0.,0.,-1.));
#29472=DIRECTION('ref_axis',(1.,0.,0.));
#29473=DIRECTION('center_axis',(0.,0.,1.));
#29474=DIRECTION('ref_axis',(1.,0.,0.));
#29475=DIRECTION('center_axis',(0.,0.,1.));
#29476=DIRECTION('ref_axis',(1.,0.,0.));
#29477=DIRECTION('',(0.,0.,1.));
#29478=DIRECTION('center_axis',(0.,0.,1.));
#29479=DIRECTION('ref_axis',(1.,0.,0.));
#29480=DIRECTION('',(0.707106781186554,8.65956056235501E-17,-0.707106781186541));
#29481=DIRECTION('center_axis',(0.,0.,-1.));
#29482=DIRECTION('ref_axis',(1.,0.,0.));
#29483=DIRECTION('center_axis',(0.,0.,1.));
#29484=DIRECTION('ref_axis',(1.,0.,0.));
#29485=DIRECTION('center_axis',(0.,0.,1.));
#29486=DIRECTION('ref_axis',(1.,0.,0.));
#29487=DIRECTION('',(0.,0.,1.));
#29488=DIRECTION('center_axis',(0.,0.,1.));
#29489=DIRECTION('ref_axis',(1.,0.,0.));
#29490=DIRECTION('',(0.707106781186554,8.65956056235501E-17,-0.707106781186541));
#29491=DIRECTION('center_axis',(0.,0.,-1.));
#29492=DIRECTION('ref_axis',(1.,0.,0.));
#29493=DIRECTION('center_axis',(0.,0.,1.));
#29494=DIRECTION('ref_axis',(1.,0.,0.));
#29495=DIRECTION('center_axis',(0.,0.,1.));
#29496=DIRECTION('ref_axis',(1.,0.,0.));
#29497=DIRECTION('',(0.,0.,1.));
#29498=DIRECTION('center_axis',(0.,-0.707106781186541,0.707106781186554));
#29499=DIRECTION('ref_axis',(1.,0.,0.));
#29500=DIRECTION('',(0.577350269189636,-0.577350269189616,-0.577350269189626));
#29501=DIRECTION('',(1.,0.,0.));
#29502=DIRECTION('',(-0.577350269189629,-0.577350269189629,-0.577350269189619));
#29503=DIRECTION('center_axis',(0.,0.707106781186541,0.707106781186554));
#29504=DIRECTION('ref_axis',(1.,0.,0.));
#29505=DIRECTION('',(-0.577350269189622,0.577350269189643,-0.577350269189612));
#29506=DIRECTION('',(-1.,0.,0.));
#29507=DIRECTION('',(-0.577350269189629,-0.577350269189629,0.577350269189619));
#29508=DIRECTION('center_axis',(-0.707106781186541,0.,0.707106781186554));
#29509=DIRECTION('ref_axis',(0.707106781186554,0.,0.707106781186541));
#29510=DIRECTION('',(0.,-1.,0.));
#29511=DIRECTION('center_axis',(0.707106781186541,0.,0.707106781186554));
#29512=DIRECTION('ref_axis',(0.707106781186554,0.,-0.707106781186541));
#29513=DIRECTION('',(0.,1.,0.));
#29514=DIRECTION('center_axis',(-1.,0.,0.));
#29515=DIRECTION('ref_axis',(0.,1.,0.));
#29516=DIRECTION('',(0.,0.,-1.));
#29517=DIRECTION('',(0.,1.,0.));
#29518=DIRECTION('',(0.,0.,-1.));
#29519=DIRECTION('center_axis',(0.,-1.,0.));
#29520=DIRECTION('ref_axis',(-1.,0.,0.));
#29521=DIRECTION('',(0.,0.,-1.));
#29522=DIRECTION('',(-1.,0.,0.));
#29523=DIRECTION('center_axis',(0.,0.923879532511296,0.382683432365067));
#29524=DIRECTION('ref_axis',(0.,-0.382683432365067,0.923879532511296));
#29525=DIRECTION('center_axis',(0.,-0.923879532511296,-0.382683432365067));
#29526=DIRECTION('ref_axis',(0.,-0.382683432365067,0.923879532511296));
#29527=DIRECTION('',(-1.,0.,0.));
#29528=DIRECTION('',(0.,-0.382683432365083,0.92387953251129));
#29529=DIRECTION('',(0.,0.38268343236507,-0.923879532511295));
#29530=DIRECTION('',(-1.,0.,0.));
#29531=DIRECTION('center_axis',(0.,0.,1.));
#29532=DIRECTION('ref_axis',(-1.,0.,0.));
#29533=DIRECTION('',(-0.38268343236509,0.,0.923879532511287));
#29534=DIRECTION('center_axis',(0.,0.,1.));
#29535=DIRECTION('ref_axis',(-1.,0.,0.));
#29536=DIRECTION('center_axis',(0.,0.,-1.));
#29537=DIRECTION('ref_axis',(-1.,0.,0.));
#29538=DIRECTION('center_axis',(0.923879532511287,0.,0.38268343236509));
#29539=DIRECTION('ref_axis',(0.38268343236509,0.,-0.923879532511287));
#29540=DIRECTION('',(-0.38268343236509,0.,0.923879532511287));
#29541=DIRECTION('',(0.,-1.,0.));
#29542=DIRECTION('',(0.,1.,0.));
#29543=DIRECTION('center_axis',(0.,0.,1.));
#29544=DIRECTION('ref_axis',(1.74550045912005E-15,1.,0.));
#29545=DIRECTION('',(0.,0.382683432365106,0.92387953251128));
#29546=DIRECTION('center_axis',(0.,0.,1.));
#29547=DIRECTION('ref_axis',(1.71569776325697E-15,1.,0.));
#29548=DIRECTION('center_axis',(0.,0.,-1.));
#29549=DIRECTION('ref_axis',(1.77635683940025E-15,1.,0.));
#29550=DIRECTION('center_axis',(0.,-0.923879532511296,0.382683432365067));
#29551=DIRECTION('ref_axis',(0.,-0.382683432365067,-0.923879532511296));
#29552=DIRECTION('center_axis',(0.,0.923879532511296,-0.382683432365067));
#29553=DIRECTION('ref_axis',(0.,0.382683432365067,0.923879532511296));
#29554=DIRECTION('',(1.,0.,0.));
#29555=DIRECTION('',(0.,0.38268343236507,0.923879532511295));
#29556=DIRECTION('',(-1.,0.,0.));
#29557=DIRECTION('',(1.,0.,0.));
#29558=DIRECTION('center_axis',(0.,0.,1.));
#29559=DIRECTION('ref_axis',(1.,1.74550045912004E-15,0.));
#29560=DIRECTION('',(0.382683432365103,0.,0.923879532511281));
#29561=DIRECTION('center_axis',(0.,0.,-1.));
#29562=DIRECTION('ref_axis',(1.,1.77635683940024E-15,0.));
#29563=DIRECTION('center_axis',(-0.923879532511286,0.,0.382683432365093));
#29564=DIRECTION('ref_axis',(0.382683432365093,0.,0.923879532511286));
#29565=DIRECTION('',(0.382683432365103,0.,0.923879532511281));
#29566=DIRECTION('',(0.,-1.,0.));
#29567=DIRECTION('center_axis',(0.,0.,1.));
#29568=DIRECTION('ref_axis',(6.98200183648019E-15,-1.,0.));
#29569=DIRECTION('center_axis',(0.,0.,-1.));
#29570=DIRECTION('ref_axis',(7.10542735760099E-15,-1.,0.));
#29571=DIRECTION('center_axis',(0.,-1.,0.));
#29572=DIRECTION('ref_axis',(-1.,0.,0.));
#29573=DIRECTION('',(0.,0.,-1.));
#29574=DIRECTION('',(1.,0.,0.));
#29575=DIRECTION('',(0.,0.,-1.));
#29576=DIRECTION('center_axis',(0.,-1.,0.));
#29577=DIRECTION('ref_axis',(0.,0.,1.));
#29578=DIRECTION('center_axis',(0.,-1.,0.));
#29579=DIRECTION('ref_axis',(0.,0.,1.));
#29580=DIRECTION('center_axis',(0.,0.,-1.));
#29581=DIRECTION('ref_axis',(7.10542735760099E-15,-1.,0.));
#29582=DIRECTION('',(0.,0.,-1.));
#29583=DIRECTION('center_axis',(0.,0.,1.));
#29584=DIRECTION('ref_axis',(0.707106781186551,-0.707106781186544,0.));
#29585=DIRECTION('center_axis',(1.,0.,0.));
#29586=DIRECTION('ref_axis',(0.,-1.,0.));
#29587=DIRECTION('',(0.,0.,-1.));
#29588=DIRECTION('',(0.,1.,0.));
#29589=DIRECTION('center_axis',(0.,0.,-1.));
#29590=DIRECTION('ref_axis',(1.,1.77635683940024E-15,0.));
#29591=DIRECTION('',(0.,0.,-1.));
#29592=DIRECTION('center_axis',(0.,0.,1.));
#29593=DIRECTION('ref_axis',(0.707106781186548,0.707106781186547,0.));
#29594=DIRECTION('center_axis',(0.,1.,0.));
#29595=DIRECTION('ref_axis',(1.,0.,0.));
#29596=DIRECTION('center_axis',(0.,1.,0.));
#29597=DIRECTION('ref_axis',(0.,0.,1.));
#29598=DIRECTION('center_axis',(0.,1.,0.));
#29599=DIRECTION('ref_axis',(0.,0.,1.));
#29600=DIRECTION('',(0.,0.,-1.));
#29601=DIRECTION('',(-1.,0.,0.));
#29602=DIRECTION('center_axis',(0.,1.,0.));
#29603=DIRECTION('ref_axis',(0.,0.,1.));
#29604=DIRECTION('',(0.,1.,0.));
#29605=DIRECTION('center_axis',(0.,-1.,0.));
#29606=DIRECTION('ref_axis',(0.,0.,1.));
#29607=DIRECTION('center_axis',(0.,-0.923879532511296,-0.382683432365067));
#29608=DIRECTION('ref_axis',(0.,-0.382683432365067,0.923879532511296));
#29609=DIRECTION('center_axis',(0.,-1.,0.));
#29610=DIRECTION('ref_axis',(0.,0.,1.));
#29611=DIRECTION('center_axis',(0.707106781186566,0.707106781186529,0.));
#29612=DIRECTION('ref_axis',(0.,0.,-1.));
#29613=DIRECTION('',(0.,0.,-1.));
#29614=DIRECTION('',(-0.357406744336602,0.357406744336621,-0.862856209461002));
#29615=DIRECTION('',(-0.357406744336583,0.357406744336602,0.862856209461017));
#29616=DIRECTION('',(0.,0.,1.));
#29617=DIRECTION('',(0.577350269189605,-0.577350269189636,0.577350269189636));
#29618=DIRECTION('center_axis',(0.707106781186566,0.,-0.707106781186529));
#29619=DIRECTION('ref_axis',(-0.707106781186529,0.,-0.707106781186566));
#29620=DIRECTION('',(0.,1.,0.));
#29621=DIRECTION('',(-0.577350269189602,-0.577350269189643,-0.577350269189633));
#29622=DIRECTION('',(0.,-1.,0.));
#29623=DIRECTION('center_axis',(0.923879532511281,0.,-0.382683432365103));
#29624=DIRECTION('ref_axis',(-0.382683432365103,0.,-0.923879532511281));
#29625=DIRECTION('',(0.,-1.,0.));
#29626=DIRECTION('',(-0.382683432365109,0.,-0.923879532511279));
#29627=DIRECTION('',(0.,1.,0.));
#29628=DIRECTION('',(-0.357406744336605,-0.357406744336599,-0.862856209461009));
#29629=DIRECTION('center_axis',(1.,0.,0.));
#29630=DIRECTION('ref_axis',(0.,1.,0.));
#29631=DIRECTION('',(0.,0.,1.));
#29632=DIRECTION('',(0.,-1.,0.));
#29633=DIRECTION('',(0.,0.,1.));
#29634=DIRECTION('',(0.,1.,0.));
#29635=DIRECTION('',(0.,0.,1.));
#29636=DIRECTION('center_axis',(0.,0.923879532511283,-0.382683432365098));
#29637=DIRECTION('ref_axis',(0.,0.382683432365098,0.923879532511283));
#29638=DIRECTION('',(-1.,0.,0.));
#29639=DIRECTION('',(-0.357406744336594,0.357406744336601,0.862856209461013));
#29640=DIRECTION('',(0.357406744336589,0.357406744336602,0.862856209461015));
#29641=DIRECTION('',(1.,0.,0.));
#29642=DIRECTION('center_axis',(-0.70710678118656,0.707106781186535,0.));
#29643=DIRECTION('ref_axis',(0.,0.,1.));
#29644=DIRECTION('',(0.357406744336593,0.357406744336606,-0.862856209461011));
#29645=DIRECTION('',(0.,0.,1.));
#29646=DIRECTION('',(0.577350269189616,0.577350269189636,-0.577350269189626));
#29647=DIRECTION('',(0.,0.,-1.));
#29648=DIRECTION('center_axis',(-0.923879532511286,0.,-0.382683432365092));
#29649=DIRECTION('ref_axis',(-0.382683432365092,0.,0.923879532511286));
#29650=DIRECTION('',(0.,-1.,0.));
#29651=DIRECTION('',(0.382683432365087,0.,-0.923879532511288));
#29652=DIRECTION('',(0.,1.,0.));
#29653=DIRECTION('center_axis',(0.,0.707106781186549,-0.707106781186546));
#29654=DIRECTION('ref_axis',(-1.,0.,0.));
#29655=DIRECTION('',(0.577350269189632,0.577350269189622,0.577350269189624));
#29656=DIRECTION('',(1.,0.,0.));
#29657=DIRECTION('',(0.577350269189629,-0.577350269189623,-0.577350269189626));
#29658=DIRECTION('center_axis',(0.,0.382683432365087,-0.923879532511288));
#29659=DIRECTION('ref_axis',(-1.,0.,0.));
#29660=DIRECTION('',(-0.357406744336593,0.862856209461018,0.357406744336591));
#29661=DIRECTION('',(-0.357406744336596,-0.862856209461017,-0.35740674433659));
#29662=DIRECTION('',(-1.,0.,0.));
#29663=DIRECTION('center_axis',(-0.707106781186546,0.,-0.707106781186549));
#29664=DIRECTION('ref_axis',(-0.707106781186549,0.,0.707106781186546));
#29665=DIRECTION('',(0.,-1.,0.));
#29666=DIRECTION('',(-0.707106781186549,-1.25607396694702E-14,0.707106781186546));
#29667=DIRECTION('center_axis',(0.,0.,-1.));
#29668=DIRECTION('ref_axis',(1.,1.83161605020261E-15,0.));
#29669=DIRECTION('',(0.923879532511282,0.,-0.382683432365102));
#29670=DIRECTION('center_axis',(1.77543178352399E-30,-9.42186760553338E-16,
1.));
#29671=DIRECTION('ref_axis',(1.,1.88437352110668E-15,0.));
#29672=DIRECTION('',(0.,-0.923879532511289,0.382683432365085));
#29673=DIRECTION('center_axis',(0.382683432365102,0.,0.923879532511282));
#29674=DIRECTION('ref_axis',(0.923879532511282,0.,-0.382683432365102));
#29675=DIRECTION('',(0.923879532511314,0.,-0.382683432365025));
#29676=DIRECTION('',(0.,1.,0.));
#29677=DIRECTION('center_axis',(0.,0.,-1.));
#29678=DIRECTION('ref_axis',(0.,-1.,0.));
#29679=DIRECTION('',(0.,-0.923879532511279,-0.38268343236511));
#29680=DIRECTION('center_axis',(4.71093380276669E-16,0.,1.));
#29681=DIRECTION('ref_axis',(0.,-1.,0.));
#29682=DIRECTION('center_axis',(0.,-0.382683432365087,0.923879532511288));
#29683=DIRECTION('ref_axis',(1.,0.,0.));
#29684=DIRECTION('',(0.,-0.923879532511279,-0.38268343236511));
#29685=DIRECTION('',(1.,0.,0.));
#29686=DIRECTION('center_axis',(0.,0.,-1.));
#29687=DIRECTION('ref_axis',(-1.,0.,0.));
#29688=DIRECTION('',(-0.923879532511282,0.,-0.382683432365102));
#29689=DIRECTION('center_axis',(0.,4.7109338027667E-16,1.));
#29690=DIRECTION('ref_axis',(-1.,0.,0.));
#29691=DIRECTION('center_axis',(-0.382683432365102,0.,0.923879532511282));
#29692=DIRECTION('ref_axis',(0.923879532511282,0.,0.382683432365102));
#29693=DIRECTION('',(-0.923879532511282,0.,-0.382683432365102));
#29694=DIRECTION('',(0.,-1.,0.));
#29695=DIRECTION('center_axis',(0.,0.,-1.));
#29696=DIRECTION('ref_axis',(9.15808025101306E-16,1.,0.));
#29697=DIRECTION('',(0.,0.923879532511285,-0.382683432365094));
#29698=DIRECTION('center_axis',(0.,0.,1.));
#29699=DIRECTION('ref_axis',(9.4218676055334E-16,1.,0.));
#29700=DIRECTION('center_axis',(0.,0.382683432365087,0.923879532511288));
#29701=DIRECTION('ref_axis',(1.,0.,0.));
#29702=DIRECTION('',(-1.,0.,0.));
#29703=DIRECTION('center_axis',(-0.707106781186548,0.,0.707106781186548));
#29704=DIRECTION('ref_axis',(0.707106781186548,0.,0.707106781186548));
#29705=DIRECTION('',(-0.707106781186548,0.,-0.707106781186548));
#29706=DIRECTION('',(0.,1.,0.));
#29707=DIRECTION('',(0.707106781186548,8.37382644631345E-15,0.707106781186548));
#29708=DIRECTION('center_axis',(0.,0.,-1.));
#29709=DIRECTION('ref_axis',(8.88178419700126E-16,1.,0.));
#29710=DIRECTION('',(0.,-0.707106781186548,0.707106781186548));
#29711=DIRECTION('center_axis',(0.,0.,-1.));
#29712=DIRECTION('ref_axis',(9.04161894879113E-16,1.,0.));
#29713=DIRECTION('center_axis',(0.,0.707106781186548,0.707106781186548));
#29714=DIRECTION('ref_axis',(1.,0.,0.));
#29715=DIRECTION('',(0.,-0.707106781186548,0.707106781186548));
#29716=DIRECTION('',(1.,0.,0.));
#29717=DIRECTION('center_axis',(0.,0.,-1.));
#29718=DIRECTION('ref_axis',(1.,1.77635683940025E-15,0.));
#29719=DIRECTION('',(-0.707106781186543,-8.3738264463135E-15,0.707106781186552));
#29720=DIRECTION('center_axis',(2.45252619645416E-30,-1.35624284231867E-15,
-1.));
#29721=DIRECTION('ref_axis',(1.,1.80832378975823E-15,0.));
#29722=DIRECTION('center_axis',(-0.923879532511287,0.,0.38268343236509));
#29723=DIRECTION('ref_axis',(0.38268343236509,0.,0.923879532511287));
#29724=DIRECTION('',(0.382683432365094,0.,0.923879532511285));
#29725=DIRECTION('',(-0.382683432365094,0.,-0.923879532511285));
#29726=DIRECTION('',(0.,-1.,0.));
#29727=DIRECTION('center_axis',(0.,0.,-1.));
#29728=DIRECTION('ref_axis',(-1.,0.,0.));
#29729=DIRECTION('',(0.,0.382683432365083,0.92387953251129));
#29730=DIRECTION('center_axis',(0.,0.,-1.));
#29731=DIRECTION('ref_axis',(-1.,0.,0.));
#29732=DIRECTION('center_axis',(0.,0.,1.));
#29733=DIRECTION('ref_axis',(-1.,0.,0.));
#29734=DIRECTION('center_axis',(0.,-0.923879532511296,0.382683432365067));
#29735=DIRECTION('ref_axis',(0.,-0.382683432365067,-0.923879532511296));
#29736=DIRECTION('center_axis',(0.,0.923879532511296,-0.382683432365067));
#29737=DIRECTION('ref_axis',(0.,0.382683432365067,0.923879532511296));
#29738=DIRECTION('',(1.,0.,0.));
#29739=DIRECTION('',(0.,0.38268343236507,0.923879532511295));
#29740=DIRECTION('',(-1.,0.,0.));
#29741=DIRECTION('',(1.,0.,0.));
#29742=DIRECTION('center_axis',(0.,0.,-1.));
#29743=DIRECTION('ref_axis',(0.,-1.,0.));
#29744=DIRECTION('',(-0.382683432365051,0.,0.923879532511303));
#29745=DIRECTION('center_axis',(-4.52080947439555E-16,0.,-1.));
#29746=DIRECTION('ref_axis',(0.,-1.,0.));
#29747=DIRECTION('center_axis',(0.,0.,1.));
#29748=DIRECTION('ref_axis',(0.,-1.,0.));
#29749=DIRECTION('center_axis',(0.923879532511273,0.,0.382683432365124));
#29750=DIRECTION('ref_axis',(0.382683432365124,0.,-0.923879532511273));
#29751=DIRECTION('',(-0.382683432365124,0.,0.923879532511273));
#29752=DIRECTION('',(0.,-1.,0.));
#29753=DIRECTION('center_axis',(0.,0.,-1.));
#29754=DIRECTION('ref_axis',(1.,1.79219777943861E-15,0.));
#29755=DIRECTION('',(0.,-0.382683432365097,0.923879532511284));
#29756=DIRECTION('center_axis',(0.,0.,1.));
#29757=DIRECTION('ref_axis',(1.,1.77635683940025E-15,0.));
#29758=DIRECTION('center_axis',(0.,0.923879532511296,0.382683432365067));
#29759=DIRECTION('ref_axis',(0.,-0.382683432365067,0.923879532511296));
#29760=DIRECTION('',(-1.,0.,0.));
#29761=DIRECTION('',(0.,-0.38268343236507,0.923879532511295));
#29762=DIRECTION('',(-1.,0.,0.));
#29763=DIRECTION('center_axis',(0.,0.,-1.));
#29764=DIRECTION('ref_axis',(8.96098889719304E-16,1.,0.));
#29765=DIRECTION('center_axis',(0.,0.,1.));
#29766=DIRECTION('ref_axis',(8.88178419700126E-16,1.,0.));
#29767=DIRECTION('center_axis',(0.,-1.,0.));
#29768=DIRECTION('ref_axis',(1.,0.,0.));
#29769=DIRECTION('',(0.,0.,1.));
#29770=DIRECTION('',(-1.,0.,0.));
#29771=DIRECTION('',(0.,0.,1.));
#29772=DIRECTION('center_axis',(0.,1.,0.));
#29773=DIRECTION('ref_axis',(0.,0.,1.));
#29774=DIRECTION('center_axis',(0.,1.,0.));
#29775=DIRECTION('ref_axis',(0.,0.,1.));
#29776=DIRECTION('center_axis',(0.,0.,1.));
#29777=DIRECTION('ref_axis',(-1.,0.,0.));
#29778=DIRECTION('',(0.,0.,1.));
#29779=DIRECTION('center_axis',(0.,0.,-1.));
#29780=DIRECTION('ref_axis',(-1.,0.,0.));
#29781=DIRECTION('center_axis',(-1.,0.,0.));
#29782=DIRECTION('ref_axis',(0.,-1.,0.));
#29783=DIRECTION('',(0.,0.,1.));
#29784=DIRECTION('',(0.,1.,0.));
#29785=DIRECTION('',(0.,0.,-1.));
#29786=DIRECTION('',(0.,1.,0.));
#29787=DIRECTION('center_axis',(0.,0.,1.));
#29788=DIRECTION('ref_axis',(8.88178419700126E-16,1.,0.));
#29789=DIRECTION('',(0.,0.,1.));
#29790=DIRECTION('center_axis',(0.,0.,-1.));
#29791=DIRECTION('ref_axis',(8.88178419700126E-16,1.,0.));
#29792=DIRECTION('center_axis',(0.,1.,0.));
#29793=DIRECTION('ref_axis',(-1.,0.,0.));
#29794=DIRECTION('',(0.,0.,1.));
#29795=DIRECTION('',(1.,0.,0.));
#29796=DIRECTION('center_axis',(0.,0.,1.));
#29797=DIRECTION('ref_axis',(0.,-1.,0.));
#29798=DIRECTION('',(0.,0.382683432365078,-0.923879532511292));
#29799=DIRECTION('center_axis',(-9.0416189487911E-16,0.,1.));
#29800=DIRECTION('ref_axis',(0.,-1.,0.));
#29801=DIRECTION('center_axis',(0.,0.,-1.));
#29802=DIRECTION('ref_axis',(0.,-1.,0.));
#29803=DIRECTION('center_axis',(0.,-0.923879532511287,-0.382683432365089));
#29804=DIRECTION('ref_axis',(0.,0.382683432365089,-0.923879532511287));
#29805=DIRECTION('',(0.,0.382683432365074,-0.923879532511293));
#29806=DIRECTION('',(1.,0.,0.));
#29807=DIRECTION('center_axis',(0.,0.,1.));
#29808=DIRECTION('ref_axis',(-1.,0.,-5.95065668954225E-17));
#29809=DIRECTION('center_axis',(-1.20084001663632E-16,3.6731576979464E-16,
1.));
#29810=DIRECTION('ref_axis',(-1.,0.,-1.20084001663632E-16));
#29811=DIRECTION('center_axis',(0.707106781186543,0.,-0.707106781186553));
#29812=DIRECTION('ref_axis',(-0.707106781186553,0.,-0.707106781186543));
#29813=DIRECTION('',(0.707106781186553,0.,0.707106781186543));
#29814=DIRECTION('',(0.,1.,0.));
#29815=DIRECTION('center_axis',(0.,0.,1.));
#29816=DIRECTION('ref_axis',(0.,-1.,0.));
#29817=DIRECTION('',(0.,-0.707106781186546,0.707106781186549));
#29818=DIRECTION('center_axis',(0.,0.,1.));
#29819=DIRECTION('ref_axis',(0.,-1.,0.));
#29820=DIRECTION('center_axis',(0.,-0.707106781186549,-0.707106781186546));
#29821=DIRECTION('ref_axis',(-1.,0.,0.));
#29822=DIRECTION('',(0.,-0.707106781186546,0.707106781186549));
#29823=DIRECTION('',(1.,0.,0.));
#29824=DIRECTION('center_axis',(0.,0.,1.));
#29825=DIRECTION('ref_axis',(-1.,0.,0.));
#29826=DIRECTION('center_axis',(0.,0.,1.));
#29827=DIRECTION('ref_axis',(-1.,0.,0.));
#29828=DIRECTION('center_axis',(0.293767845955579,-0.29376784595556,-0.909615800965028));
#29829=DIRECTION('ref_axis',(-0.951603598919524,0.,-0.307328147951679));
#29830=DIRECTION('',(0.252587513646048,-0.893921863713326,0.37027455965189));
#29831=DIRECTION('',(-0.893921863713342,0.252587513646,-0.370274559651883));
#29832=DIRECTION('',(0.707106781186522,0.707106781186573,-2.56395024851135E-15));
#29833=DIRECTION('center_axis',(-0.293767845955583,-0.293767845955567,-0.909615800965025));
#29834=DIRECTION('ref_axis',(-0.951603598919523,0.,0.307328147951684));
#29835=DIRECTION('',(0.707106781186537,-0.707106781186558,-2.05116019880918E-14));
#29836=DIRECTION('',(-0.893921863713315,-0.252587513646067,0.370274559651903));
#29837=DIRECTION('',(0.252587513646048,0.893921863713326,-0.37027455965189));
#29838=DIRECTION('center_axis',(0.382683432365075,0.,-0.923879532511293));
#29839=DIRECTION('ref_axis',(-0.923879532511293,0.,-0.382683432365075));
#29840=DIRECTION('',(0.923879532511287,1.92271478790291E-14,0.38268343236509));
#29841=DIRECTION('',(0.,-1.,0.));
#29842=DIRECTION('',(0.,1.,0.));
#29843=DIRECTION('center_axis',(0.,0.,1.));
#29844=DIRECTION('ref_axis',(1.,1.80669269305388E-15,0.));
#29845=DIRECTION('',(0.,0.923879532511307,0.382683432365042));
#29846=DIRECTION('center_axis',(6.58156273757651E-32,-3.58533327904521E-17,
-1.));
#29847=DIRECTION('ref_axis',(1.,1.83569063887115E-15,0.));
#29848=DIRECTION('center_axis',(0.,0.,1.));
#29849=DIRECTION('ref_axis',(1.,1.77635683940025E-15,0.));
#29850=DIRECTION('center_axis',(0.,0.382683432365087,-0.923879532511288));
#29851=DIRECTION('ref_axis',(-1.,0.,0.));
#29852=DIRECTION('',(0.,0.923879532511291,0.382683432365079));
#29853=DIRECTION('',(1.,0.,0.));
#29854=DIRECTION('',(-1.,0.,0.));
#29855=DIRECTION('center_axis',(0.,0.,1.));
#29856=DIRECTION('ref_axis',(9.03346346526939E-16,1.,0.));
#29857=DIRECTION('',(-0.923879532511288,0.,0.382683432365088));
#29858=DIRECTION('center_axis',(2.40217329696029E-16,-2.20482351708812E-31,
-1.));
#29859=DIRECTION('ref_axis',(9.17845319435574E-16,1.,0.));
#29860=DIRECTION('center_axis',(0.,0.,1.));
#29861=DIRECTION('ref_axis',(8.88178419700126E-16,1.,0.));
#29862=DIRECTION('center_axis',(-0.382683432365103,0.,-0.923879532511281));
#29863=DIRECTION('ref_axis',(-0.923879532511281,0.,0.382683432365103));
#29864=DIRECTION('',(0.,-1.,0.));
#29865=DIRECTION('',(0.,1.,0.));
#29866=DIRECTION('center_axis',(0.,-0.382683432365087,-0.923879532511288));
#29867=DIRECTION('ref_axis',(-1.,0.,0.));
#29868=DIRECTION('',(-1.,0.,0.));
#29869=DIRECTION('',(1.,0.,0.));
#29870=DIRECTION('center_axis',(0.585030164998638,-0.585030164998597,-0.56167553986566));
#29871=DIRECTION('ref_axis',(-0.692561717404368,0.,-0.721358626194982));
#29872=DIRECTION('',(0.707106781186527,0.707106781186568,5.12790049702273E-15));
#29873=DIRECTION('',(0.341690748410332,-0.450292794593974,0.824914438949602));
#29874=DIRECTION('',(-0.707106781186522,-0.707106781186573,-2.70840949122957E-14));
#29875=DIRECTION('',(-0.450292794593978,0.341690748410326,-0.824914438949602));
#29876=DIRECTION('center_axis',(-0.585030164998638,-0.585030164998608,-0.561675539865649));
#29877=DIRECTION('ref_axis',(-0.692561717404361,0.,0.721358626194989));
#29878=DIRECTION('',(-0.450292794593951,-0.341690748410332,0.824914438949615));
#29879=DIRECTION('',(-0.707106781186541,0.707106781186554,1.37383090134832E-14));
#29880=DIRECTION('',(0.341690748410326,0.450292794593954,-0.824914438949615));
#29881=DIRECTION('',(0.707106781186553,-0.707106781186542,-2.5639502485115E-14));
#29882=DIRECTION('center_axis',(-0.707106781186554,-0.707106781186541,0.));
#29883=DIRECTION('ref_axis',(0.,0.,1.));
#29884=DIRECTION('',(0.,0.,1.));
#29885=DIRECTION('',(-0.577350269189605,0.577350269189636,0.577350269189636));
#29886=DIRECTION('center_axis',(-0.707106781186541,0.,-0.707106781186554));
#29887=DIRECTION('ref_axis',(-0.707106781186554,0.,0.707106781186541));
#29888=DIRECTION('',(0.,-1.,0.));
#29889=DIRECTION('center_axis',(-0.923879532511286,0.,-0.382683432365092));
#29890=DIRECTION('ref_axis',(-0.382683432365092,0.,0.923879532511286));
#29891=DIRECTION('',(0.382683432365091,0.,-0.923879532511286));
#29892=DIRECTION('',(0.,-1.,0.));
#29893=DIRECTION('center_axis',(0.,0.,1.));
#29894=DIRECTION('ref_axis',(8.96098889719304E-16,1.,0.));
#29895=DIRECTION('',(0.,-0.382683432365091,-0.923879532511287));
#29896=DIRECTION('center_axis',(0.,0.,1.));
#29897=DIRECTION('ref_axis',(9.04161894879114E-16,1.,0.));
#29898=DIRECTION('center_axis',(0.,0.923879532511287,-0.382683432365089));
#29899=DIRECTION('ref_axis',(0.,0.382683432365089,0.923879532511287));
#29900=DIRECTION('',(0.,-0.382683432365091,-0.923879532511286));
#29901=DIRECTION('',(-1.,0.,0.));
#29902=DIRECTION('center_axis',(0.,0.,1.));
#29903=DIRECTION('ref_axis',(1.,1.79219777943861E-15,0.));
#29904=DIRECTION('',(-0.382683432365101,0.,-0.923879532511282));
#29905=DIRECTION('center_axis',(1.72443248188183E-30,-9.53608248505313E-16,
1.));
#29906=DIRECTION('ref_axis',(1.,1.80832378975823E-15,0.));
#29907=DIRECTION('center_axis',(0.,0.,-1.));
#29908=DIRECTION('ref_axis',(1.,1.77635683940025E-15,0.));
#29909=DIRECTION('center_axis',(0.923879532511281,0.,-0.382683432365103));
#29910=DIRECTION('ref_axis',(-0.382683432365103,0.,-0.923879532511281));
#29911=DIRECTION('',(0.,1.,0.));
#29912=DIRECTION('center_axis',(-0.408248290463875,-0.408248290463851,-0.816496580927726));
#29913=DIRECTION('ref_axis',(-0.894427190999911,0.,0.447213595499968));
#29914=DIRECTION('',(-0.577350269189629,-0.577350269189623,0.577350269189626));
#29915=DIRECTION('',(0.577350269189629,0.577350269189623,-0.577350269189626));
#29916=DIRECTION('center_axis',(0.,-0.923879532511283,-0.382683432365098));
#29917=DIRECTION('ref_axis',(0.,0.382683432365098,-0.923879532511283));
#29918=DIRECTION('',(1.,0.,0.));
#29919=DIRECTION('',(-1.,0.,0.));
#29920=DIRECTION('center_axis',(0.707106781186573,-0.707106781186522,0.));
#29921=DIRECTION('ref_axis',(0.,0.,-1.));
#29922=DIRECTION('',(0.,0.,-1.));
#29923=DIRECTION('center_axis',(0.408248290463882,-0.408248290463841,-0.816496580927727));
#29924=DIRECTION('ref_axis',(-0.894427190999908,0.,-0.447213595499974));
#29925=DIRECTION('',(0.577350269189632,-0.577350269189622,0.577350269189624));
#29926=DIRECTION('',(-0.577350269189632,0.577350269189622,-0.577350269189624));
#29927=DIRECTION('center_axis',(0.,0.,1.));
#29928=DIRECTION('ref_axis',(1.,1.77635683940025E-15,0.));
#29929=DIRECTION('',(0.,0.707106781186565,0.70710678118653));
#29930=DIRECTION('',(0.707106781186553,1.25607396694701E-14,0.707106781186543));
#29931=DIRECTION('center_axis',(-0.707106781186546,0.,-0.707106781186549));
#29932=DIRECTION('ref_axis',(-0.707106781186549,0.,0.707106781186546));
#29933=DIRECTION('',(-0.707106781186546,0.,0.707106781186549));
#29934=DIRECTION('center_axis',(0.,0.707106781186549,-0.707106781186546));
#29935=DIRECTION('ref_axis',(-1.,0.,0.));
#29936=DIRECTION('',(0.,0.707106781186546,0.707106781186549));
#29937=DIRECTION('center_axis',(0.,0.,1.));
#29938=DIRECTION('ref_axis',(8.88178419700126E-16,1.,0.));
#29939=DIRECTION('center_axis',(0.,-1.,0.));
#29940=DIRECTION('ref_axis',(1.,0.,0.));
#29941=DIRECTION('',(1.,0.,0.));
#29942=DIRECTION('center_axis',(0.,0.,1.));
#29943=DIRECTION('ref_axis',(1.,0.,0.));
#29944=DIRECTION('',(-1.,0.,0.));
#29945=DIRECTION('center_axis',(0.,0.,1.));
#29946=DIRECTION('ref_axis',(1.,0.,0.));
#29947=DIRECTION('center_axis',(0.,1.,0.));
#29948=DIRECTION('ref_axis',(-1.,0.,0.));
#29949=DIRECTION('center_axis',(0.,0.,1.));
#29950=DIRECTION('ref_axis',(1.,0.,0.));
#29951=DIRECTION('center_axis',(0.,-0.707106781186549,-0.707106781186546));
#29952=DIRECTION('ref_axis',(-1.,0.,0.));
#29953=DIRECTION('center_axis',(0.707106781186543,0.,-0.707106781186553));
#29954=DIRECTION('ref_axis',(-0.707106781186553,0.,-0.707106781186543));
#29955=DIRECTION('center_axis',(0.,0.,1.));
#29956=DIRECTION('ref_axis',(1.,0.,0.));
#29957=DIRECTION('center_axis',(0.,0.,-1.));
#29958=DIRECTION('ref_axis',(-1.,0.,0.));
#29959=DIRECTION('center_axis',(0.,-1.,0.));
#29960=DIRECTION('ref_axis',(-1.,0.,0.));
#29961=DIRECTION('center_axis',(1.,0.,0.));
#29962=DIRECTION('ref_axis',(0.,0.,-1.));
#29963=DIRECTION('center_axis',(0.,0.,1.));
#29964=DIRECTION('ref_axis',(-0.707106781186547,0.707106781186548,0.));
#29965=DIRECTION('center_axis',(1.,0.,0.));
#29966=DIRECTION('ref_axis',(0.,0.707106781186547,-0.707106781186547));
#29967=DIRECTION('center_axis',(1.,0.,0.));
#29968=DIRECTION('ref_axis',(0.,0.,-1.));
#29969=DIRECTION('center_axis',(0.,0.,-1.));
#29970=DIRECTION('ref_axis',(-1.,0.,0.));
#29971=DIRECTION('center_axis',(0.,-1.,0.));
#29972=DIRECTION('ref_axis',(0.,0.,-1.));
#29973=DIRECTION('center_axis',(0.,-1.,0.));
#29974=DIRECTION('ref_axis',(0.707106781186543,0.,-0.707106781186552));
#29975=DIRECTION('center_axis',(-5.92118946466756E-15,-1.,0.));
#29976=DIRECTION('ref_axis',(0.,0.,-1.));
#29977=DIRECTION('center_axis',(0.,0.,-1.));
#29978=DIRECTION('ref_axis',(-1.,0.,0.));
#29979=DIRECTION('center_axis',(-1.,-2.368475785867E-14,0.));
#29980=DIRECTION('ref_axis',(0.,0.,-1.));
#29981=DIRECTION('center_axis',(-1.,0.,0.));
#29982=DIRECTION('ref_axis',(0.,-0.707106781186547,-0.707106781186547));
#29983=DIRECTION('center_axis',(-1.,5.92118946466752E-15,0.));
#29984=DIRECTION('ref_axis',(0.,0.,-1.));
#29985=DIRECTION('center_axis',(0.,0.,-1.));
#29986=DIRECTION('ref_axis',(-1.,0.,0.));
#29987=DIRECTION('center_axis',(0.,1.,0.));
#29988=DIRECTION('ref_axis',(0.,0.,-1.));
#29989=DIRECTION('center_axis',(0.,0.,1.));
#29990=DIRECTION('ref_axis',(-0.707106781186548,-0.707106781186548,0.));
#29991=DIRECTION('center_axis',(0.,1.,0.));
#29992=DIRECTION('ref_axis',(-0.707106781186552,0.,-0.707106781186543));
#29993=DIRECTION('',(0.,-1.,0.));
#29994=DIRECTION('center_axis',(0.,0.,-1.));
#29995=DIRECTION('ref_axis',(-1.,0.,0.));
#29996=DIRECTION('',(0.,0.,-1.));
#29997=DIRECTION('center_axis',(-1.,0.,0.));
#29998=DIRECTION('ref_axis',(0.,1.,0.));
#29999=DIRECTION('',(0.,0.,-1.));
#30000=DIRECTION('center_axis',(0.,0.,-1.));
#30001=DIRECTION('ref_axis',(1.77635683940025E-15,1.,0.));
#30002=DIRECTION('center_axis',(0.,0.,1.));
#30003=DIRECTION('ref_axis',(-1.,0.,0.));
#30004=DIRECTION('',(-0.707106781186548,0.,0.707106781186548));
#30005=DIRECTION('center_axis',(0.707106781186543,0.,0.707106781186552));
#30006=DIRECTION('ref_axis',(0.707106781186552,0.,-0.707106781186543));
#30007=DIRECTION('',(-0.707106781186552,0.,0.707106781186543));
#30008=DIRECTION('center_axis',(0.,0.,1.));
#30009=DIRECTION('ref_axis',(1.77635683940025E-15,1.,0.));
#30010=DIRECTION('',(0.,0.707106781186548,0.707106781186548));
#30011=DIRECTION('center_axis',(0.,-0.707106781186548,0.707106781186548));
#30012=DIRECTION('ref_axis',(1.,0.,0.));
#30013=DIRECTION('center_axis',(0.,0.,-1.));
#30014=DIRECTION('ref_axis',(-1.,0.,0.));
#30015=DIRECTION('',(0.,0.707106781186548,0.707106781186548));
#30016=DIRECTION('center_axis',(0.,-0.707106781186548,0.707106781186548));
#30017=DIRECTION('ref_axis',(1.,0.,0.));
#30018=DIRECTION('',(0.,0.707106781186548,0.707106781186548));
#30019=DIRECTION('center_axis',(0.,0.,-1.));
#30020=DIRECTION('ref_axis',(0.,-1.,0.));
#30021=DIRECTION('',(-0.707106781186527,0.,0.707106781186568));
#30022=DIRECTION('center_axis',(0.707106781186552,0.,0.707106781186543));
#30023=DIRECTION('ref_axis',(0.707106781186543,0.,-0.707106781186552));
#30024=DIRECTION('center_axis',(0.,0.,1.));
#30025=DIRECTION('ref_axis',(0.,-1.,0.));
#30026=DIRECTION('center_axis',(0.,1.,0.));
#30027=DIRECTION('ref_axis',(0.,0.,1.));
#30028=DIRECTION('',(0.,1.,0.));
#30029=DIRECTION('center_axis',(0.,0.,1.));
#30030=DIRECTION('ref_axis',(1.,0.,0.));
#30031=DIRECTION('',(0.,0.,1.));
#30032=DIRECTION('center_axis',(0.,0.,1.));
#30033=DIRECTION('ref_axis',(1.,0.,0.));
#30034=DIRECTION('',(-0.857167300702113,-1.04972719113862E-16,0.515038074910052));
#30035=DIRECTION('center_axis',(0.,0.,1.));
#30036=DIRECTION('ref_axis',(1.,0.,0.));
#30037=DIRECTION('',(-0.857167300702113,-1.04972719113862E-16,0.515038074910052));
#30038=DIRECTION('center_axis',(0.,0.,1.));
#30039=DIRECTION('ref_axis',(1.,0.,0.));
#30040=DIRECTION('',(-0.857167300702112,-1.04972719113862E-16,0.515038074910055));
#30041=DIRECTION('center_axis',(0.,0.,1.));
#30042=DIRECTION('ref_axis',(1.,0.,0.));
#30043=DIRECTION('',(-0.857167300702112,-1.04972719113862E-16,0.515038074910055));
#30044=DIRECTION('center_axis',(1.,0.,0.));
#30045=DIRECTION('ref_axis',(0.,-1.,0.));
#30046=DIRECTION('',(0.,0.,-1.));
#30047=DIRECTION('',(0.,-1.,0.));
#30048=DIRECTION('center_axis',(0.,1.,0.));
#30049=DIRECTION('ref_axis',(1.,0.,0.));
#30050=DIRECTION('',(1.,0.,0.));
#30051=DIRECTION('center_axis',(0.,0.,-1.));
#30052=DIRECTION('ref_axis',(-1.,0.,0.));
#30053=DIRECTION('center_axis',(0.,0.,1.));
#30054=DIRECTION('ref_axis',(1.,1.77635683940025E-15,0.));
#36382=CARTESIAN_POINT('',(0.,0.,0.));
#36383=CARTESIAN_POINT('Origin',(34.6,13.,5.98232233047034));
#36384=CARTESIAN_POINT('',(34.6,14.2,6.));
#36385=CARTESIAN_POINT('',(34.6,14.1146446609407,5.96464466094067));
#36386=CARTESIAN_POINT('',(34.6,14.2,6.));
#36387=CARTESIAN_POINT('',(35.7146446609407,13.,5.96464466094067));
#36388=CARTESIAN_POINT('Origin',(34.6,13.,5.96464466094067));
#36389=CARTESIAN_POINT('',(35.8,13.,6.));
#36390=CARTESIAN_POINT('',(35.7146446609407,13.,5.96464466094067));
#36391=CARTESIAN_POINT('Origin',(34.6,13.,6.));
#36392=CARTESIAN_POINT('Origin',(18.85,14.1573223304703,5.98232233047034));
#36393=CARTESIAN_POINT('',(9.4,14.2,6.));
#36394=CARTESIAN_POINT('',(9.4,14.1146446609407,5.96464466094067));
#36395=CARTESIAN_POINT('',(9.4,14.2,6.));
#36396=CARTESIAN_POINT('',(18.85,14.1146446609407,5.96464466094067));
#36397=CARTESIAN_POINT('',(18.85,14.2,6.));
#36398=CARTESIAN_POINT('Origin',(9.4,13.,5.98232233047034));
#36399=CARTESIAN_POINT('',(8.2,13.,6.));
#36400=CARTESIAN_POINT('',(8.28535533905933,13.,5.96464466094067));
#36401=CARTESIAN_POINT('',(8.2,13.,6.));
#36402=CARTESIAN_POINT('Origin',(9.4,13.,5.96464466094067));
#36403=CARTESIAN_POINT('Origin',(9.4,13.,6.));
#36404=CARTESIAN_POINT('Origin',(8.24267766952966,-3.25,5.98232233047034));
#36405=CARTESIAN_POINT('',(8.2,-13.,6.));
#36406=CARTESIAN_POINT('',(8.28535533905933,-13.,5.96464466094067));
#36407=CARTESIAN_POINT('',(8.2,-13.,6.));
#36408=CARTESIAN_POINT('',(8.28535533905933,-3.25,5.96464466094067));
#36409=CARTESIAN_POINT('',(8.2,-3.25,6.));
#36410=CARTESIAN_POINT('Origin',(9.4,-13.,5.98232233047034));
#36411=CARTESIAN_POINT('',(9.4,-14.2,6.));
#36412=CARTESIAN_POINT('',(9.4,-14.1146446609407,5.96464466094067));
#36413=CARTESIAN_POINT('',(9.4,-14.2,6.));
#36414=CARTESIAN_POINT('Origin',(9.4,-13.,5.96464466094067));
#36415=CARTESIAN_POINT('Origin',(9.4,-13.,6.));
#36416=CARTESIAN_POINT('Origin',(25.15,-14.1573223304703,5.98232233047034));
#36417=CARTESIAN_POINT('',(34.6,-14.2,6.));
#36418=CARTESIAN_POINT('',(34.6,-14.1146446609407,5.96464466094067));
#36419=CARTESIAN_POINT('',(34.6,-14.2,6.));
#36420=CARTESIAN_POINT('',(25.15,-14.1146446609407,5.96464466094067));
#36421=CARTESIAN_POINT('',(25.15,-14.2,6.));
#36422=CARTESIAN_POINT('Origin',(34.6,-13.,5.98232233047034));
#36423=CARTESIAN_POINT('',(35.8,-13.,6.));
#36424=CARTESIAN_POINT('',(35.7146446609407,-13.,5.96464466094067));
#36425=CARTESIAN_POINT('',(35.8,-13.,6.));
#36426=CARTESIAN_POINT('Origin',(34.6,-13.,5.96464466094067));
#36427=CARTESIAN_POINT('Origin',(34.6,-13.,6.));
#36428=CARTESIAN_POINT('Origin',(35.7573223304703,3.25,5.98232233047034));
#36429=CARTESIAN_POINT('',(35.7146446609407,3.25,5.96464466094067));
#36430=CARTESIAN_POINT('',(35.8,3.25,6.));
#36431=CARTESIAN_POINT('Origin',(28.3,-14.075,5.925));
#36432=CARTESIAN_POINT('',(34.6,-14.0353553390593,5.88535533905933));
#36433=CARTESIAN_POINT('',(34.6,-14.15,6.));
#36434=CARTESIAN_POINT('',(9.4,-14.0353553390593,5.88535533905933));
#36435=CARTESIAN_POINT('',(31.45,-14.0353553390593,5.88535533905933));
#36436=CARTESIAN_POINT('',(9.4,-14.,5.85));
#36437=CARTESIAN_POINT('Origin',(34.6,-13.,5.925));
#36438=CARTESIAN_POINT('',(35.6353553390593,-13.,5.88535533905933));
#36439=CARTESIAN_POINT('',(35.6,-13.,5.85));
#36440=CARTESIAN_POINT('Origin',(34.6,-13.,5.88535533905933));
#36441=CARTESIAN_POINT('Origin',(35.675,6.5,5.925));
#36442=CARTESIAN_POINT('',(35.6353553390593,13.,5.88535533905933));
#36443=CARTESIAN_POINT('',(35.6,13.,5.85));
#36444=CARTESIAN_POINT('',(35.6353553390593,9.75,5.88535533905933));
#36445=CARTESIAN_POINT('Origin',(34.6,13.,5.925));
#36446=CARTESIAN_POINT('',(34.6,14.0353553390593,5.88535533905933));
#36447=CARTESIAN_POINT('',(34.6,14.,5.85));
#36448=CARTESIAN_POINT('Origin',(34.6,13.,5.88535533905933));
#36449=CARTESIAN_POINT('Origin',(22.,0.,6.));
#36450=CARTESIAN_POINT('',(35.,15.,6.));
#36451=CARTESIAN_POINT('',(36.8,13.2,6.));
#36452=CARTESIAN_POINT('Origin',(35.,13.2,6.));
#36453=CARTESIAN_POINT('',(9.,15.,6.));
#36454=CARTESIAN_POINT('',(25.25,15.,6.));
#36455=CARTESIAN_POINT('',(7.2,13.2,6.));
#36456=CARTESIAN_POINT('Origin',(9.,13.2,6.));
#36457=CARTESIAN_POINT('',(7.2,-13.2,6.));
#36458=CARTESIAN_POINT('',(7.2,3.3,6.));
#36459=CARTESIAN_POINT('',(9.,-15.,6.));
#36460=CARTESIAN_POINT('Origin',(9.,-13.2,6.));
#36461=CARTESIAN_POINT('',(35.,-15.,6.));
#36462=CARTESIAN_POINT('',(18.75,-15.,6.));
#36463=CARTESIAN_POINT('',(36.8,-13.2,6.));
#36464=CARTESIAN_POINT('Origin',(35.,-13.2,6.));
#36465=CARTESIAN_POINT('',(36.8,-3.3,6.));
#36466=CARTESIAN_POINT('Origin',(29.,-9.2,4.175));
#36467=CARTESIAN_POINT('',(28.445,-9.2,4.2));
#36468=CARTESIAN_POINT('Origin',(29.,-9.2,4.2));
#36469=CARTESIAN_POINT('',(28.495,-9.2,4.15));
#36470=CARTESIAN_POINT('',(28.47,-9.2,4.175));
#36471=CARTESIAN_POINT('Origin',(29.,-9.2,4.15));
#36472=CARTESIAN_POINT('Origin',(22.,3.5527136788005E-15,4.2));
#36473=CARTESIAN_POINT('',(8.7,13.,4.2));
#36474=CARTESIAN_POINT('',(9.4,13.7,4.2));
#36475=CARTESIAN_POINT('Origin',(9.4,13.,4.2));
#36476=CARTESIAN_POINT('',(8.7,-13.,4.2));
#36477=CARTESIAN_POINT('',(8.7,-6.5,4.2));
#36478=CARTESIAN_POINT('',(9.4,-13.7,4.2));
#36479=CARTESIAN_POINT('Origin',(9.4,-13.,4.2));
#36480=CARTESIAN_POINT('',(34.6,-13.7,4.2));
#36481=CARTESIAN_POINT('',(28.3,-13.7,4.2));
#36482=CARTESIAN_POINT('',(35.3,-13.,4.2));
#36483=CARTESIAN_POINT('Origin',(34.6,-13.,4.2));
#36484=CARTESIAN_POINT('',(35.3,13.,4.2));
#36485=CARTESIAN_POINT('',(35.3,6.5,4.2));
#36486=CARTESIAN_POINT('',(34.6,13.7,4.2));
#36487=CARTESIAN_POINT('Origin',(34.6,13.,4.2));
#36488=CARTESIAN_POINT('',(15.7,13.7,4.2));
#36489=CARTESIAN_POINT('',(28.445,9.2,4.2));
#36490=CARTESIAN_POINT('Origin',(29.,9.2,4.2));
#36491=CARTESIAN_POINT('',(10.445,9.2,4.2));
#36492=CARTESIAN_POINT('Origin',(11.,9.2,4.2));
#36493=CARTESIAN_POINT('',(32.725,1.07156594925393E-16,4.2));
#36494=CARTESIAN_POINT('Origin',(33.6,0.,4.2));
#36495=CARTESIAN_POINT('',(18.95,-12.55,4.2));
#36496=CARTESIAN_POINT('',(21.05,-12.55,4.2));
#36497=CARTESIAN_POINT('',(21.5,-12.55,4.2));
#36498=CARTESIAN_POINT('',(18.95,12.55,4.2));
#36499=CARTESIAN_POINT('',(18.95,-6.25,4.2));
#36500=CARTESIAN_POINT('',(21.05,12.55,4.2));
#36501=CARTESIAN_POINT('',(20.5,12.55,4.2));
#36502=CARTESIAN_POINT('',(21.05,6.25,4.2));
#36503=CARTESIAN_POINT('',(10.445,-9.2,4.2));
#36504=CARTESIAN_POINT('Origin',(11.,-9.2,4.2));
#36505=CARTESIAN_POINT('Origin',(29.,-9.2,3.215));
#36506=CARTESIAN_POINT('',(28.495,-9.2,2.2));
#36507=CARTESIAN_POINT('Origin',(29.,-9.2,2.2));
#36508=CARTESIAN_POINT('',(28.495,-9.2,3.215));
#36509=CARTESIAN_POINT('Origin',(29.,9.2,4.175));
#36510=CARTESIAN_POINT('',(28.495,9.2,4.15));
#36511=CARTESIAN_POINT('',(28.47,9.2,4.175));
#36512=CARTESIAN_POINT('Origin',(29.,9.2,4.15));
#36513=CARTESIAN_POINT('Origin',(29.,9.2,3.215));
#36514=CARTESIAN_POINT('',(28.495,9.2,2.2));
#36515=CARTESIAN_POINT('Origin',(29.,9.2,2.2));
#36516=CARTESIAN_POINT('',(28.495,9.2,3.215));
#36517=CARTESIAN_POINT('Origin',(11.,-9.2,4.175));
#36518=CARTESIAN_POINT('',(10.495,-9.2,4.15));
#36519=CARTESIAN_POINT('',(10.47,-9.2,4.175));
#36520=CARTESIAN_POINT('Origin',(11.,-9.2,4.15));
#36521=CARTESIAN_POINT('Origin',(11.,-9.2,3.215));
#36522=CARTESIAN_POINT('',(10.495,-9.2,2.2));
#36523=CARTESIAN_POINT('Origin',(11.,-9.2,2.2));
#36524=CARTESIAN_POINT('',(10.495,-9.2,3.215));
#36525=CARTESIAN_POINT('Origin',(11.,9.2,4.175));
#36526=CARTESIAN_POINT('',(10.495,9.2,4.15));
#36527=CARTESIAN_POINT('',(10.47,9.2,4.175));
#36528=CARTESIAN_POINT('Origin',(11.,9.2,4.15));
#36529=CARTESIAN_POINT('Origin',(11.,9.2,3.215));
#36530=CARTESIAN_POINT('',(10.495,9.2,2.2));
#36531=CARTESIAN_POINT('Origin',(11.,9.2,2.2));
#36532=CARTESIAN_POINT('',(10.495,9.2,3.215));
#36533=CARTESIAN_POINT('Origin',(20.5,12.525,4.175));
#36534=CARTESIAN_POINT('',(19.,12.5,4.15));
#36535=CARTESIAN_POINT('',(18.95,12.55,4.2));
#36536=CARTESIAN_POINT('',(21.,12.5,4.15));
#36537=CARTESIAN_POINT('',(20.5,12.5,4.15));
#36538=CARTESIAN_POINT('',(21.05,12.55,4.2));
#36539=CARTESIAN_POINT('Origin',(21.5,-12.525,4.175));
#36540=CARTESIAN_POINT('',(21.,-12.5,4.15));
#36541=CARTESIAN_POINT('',(21.05,-12.55,4.2));
#36542=CARTESIAN_POINT('',(19.,-12.5,4.15));
#36543=CARTESIAN_POINT('',(21.5,-12.5,4.15));
#36544=CARTESIAN_POINT('',(19.,-12.5,4.15));
#36545=CARTESIAN_POINT('Origin',(21.025,6.25,4.175));
#36546=CARTESIAN_POINT('',(21.,6.25,4.15));
#36547=CARTESIAN_POINT('Origin',(18.975,-6.25,4.175));
#36548=CARTESIAN_POINT('',(19.,-6.25,4.15));
#36549=CARTESIAN_POINT('Origin',(19.,-12.5,4.2));
#36550=CARTESIAN_POINT('',(19.,-12.5,3.6));
#36551=CARTESIAN_POINT('',(19.,-12.5,4.2));
#36552=CARTESIAN_POINT('',(19.,12.5,3.6));
#36553=CARTESIAN_POINT('',(19.,12.5,3.6));
#36554=CARTESIAN_POINT('',(19.,12.5,4.2));
#36555=CARTESIAN_POINT('Origin',(21.,-12.5,4.2));
#36556=CARTESIAN_POINT('',(21.,-12.5,3.6));
#36557=CARTESIAN_POINT('',(21.,-12.5,4.2));
#36558=CARTESIAN_POINT('',(19.,-12.5,3.6));
#36559=CARTESIAN_POINT('Origin',(31.45,-14.0176776695297,5.84267766952966));
#36560=CARTESIAN_POINT('',(20.0776208734813,-14.,5.8));
#36561=CARTESIAN_POINT('',(19.9223791265187,-14.,5.8));
#36562=CARTESIAN_POINT('Origin',(20.,-13.7514718625762,5.2));
#36563=CARTESIAN_POINT('',(9.4,-14.,5.8));
#36564=CARTESIAN_POINT('',(31.45,-14.,5.8));
#36565=CARTESIAN_POINT('',(9.4,-14.,5.8));
#36566=CARTESIAN_POINT('',(34.6,-14.,5.8));
#36567=CARTESIAN_POINT('',(34.6,-14.0353553390593,5.88535533905933));
#36568=CARTESIAN_POINT('',(31.45,-14.,5.8));
#36569=CARTESIAN_POINT('Origin',(9.4,-13.,5.84267766952966));
#36570=CARTESIAN_POINT('',(8.4,-13.,5.8));
#36571=CARTESIAN_POINT('',(8.36464466094067,-13.,5.88535533905933));
#36572=CARTESIAN_POINT('',(8.4,-13.,5.8));
#36573=CARTESIAN_POINT('Origin',(9.4,-13.,5.88535533905933));
#36574=CARTESIAN_POINT('Origin',(9.4,-13.,5.8));
#36575=CARTESIAN_POINT('Origin',(8.38232233047034,-9.75,5.84267766952966));
#36576=CARTESIAN_POINT('',(8.4,13.,5.8));
#36577=CARTESIAN_POINT('',(8.36464466094067,13.,5.88535533905933));
#36578=CARTESIAN_POINT('',(8.4,13.,5.8));
#36579=CARTESIAN_POINT('',(8.36464466094067,-9.75,5.88535533905933));
#36580=CARTESIAN_POINT('',(8.4,-9.75,5.8));
#36581=CARTESIAN_POINT('Origin',(9.4,13.,5.84267766952966));
#36582=CARTESIAN_POINT('',(9.4,14.,5.8));
#36583=CARTESIAN_POINT('',(9.4,14.0353553390593,5.88535533905933));
#36584=CARTESIAN_POINT('',(9.4,14.,5.8));
#36585=CARTESIAN_POINT('Origin',(9.4,13.,5.88535533905933));
#36586=CARTESIAN_POINT('Origin',(9.4,13.,5.8));
#36587=CARTESIAN_POINT('Origin',(12.55,14.0176776695297,5.84267766952966));
#36588=CARTESIAN_POINT('',(19.9223791265187,14.,5.8));
#36589=CARTESIAN_POINT('',(20.0776208734813,14.,5.8));
#36590=CARTESIAN_POINT('Origin',(20.,13.7514718625762,5.2));
#36591=CARTESIAN_POINT('',(34.6,14.,5.8));
#36592=CARTESIAN_POINT('',(12.55,14.,5.8));
#36593=CARTESIAN_POINT('',(34.6,14.,5.8));
#36594=CARTESIAN_POINT('',(12.55,14.0353553390593,5.88535533905933));
#36595=CARTESIAN_POINT('',(12.55,14.,5.8));
#36596=CARTESIAN_POINT('Origin',(34.6,13.,5.84267766952966));
#36597=CARTESIAN_POINT('',(35.6,13.,5.8));
#36598=CARTESIAN_POINT('',(35.6,13.,5.8));
#36599=CARTESIAN_POINT('Origin',(34.6,13.,5.8));
#36600=CARTESIAN_POINT('Origin',(35.6176776695297,9.75,5.84267766952967));
#36601=CARTESIAN_POINT('',(35.6,-13.,5.8));
#36602=CARTESIAN_POINT('',(35.6,-13.,5.8));
#36603=CARTESIAN_POINT('',(35.6,9.75,5.8));
#36604=CARTESIAN_POINT('Origin',(34.6,-13.,5.84267766952966));
#36605=CARTESIAN_POINT('Origin',(34.6,-13.,5.8));
#36606=CARTESIAN_POINT('Origin',(34.6,-14.,6.));
#36607=CARTESIAN_POINT('',(34.6,-14.,4.5));
#36608=CARTESIAN_POINT('',(34.6,-14.,6.));
#36609=CARTESIAN_POINT('',(9.4,-14.,4.5));
#36610=CARTESIAN_POINT('',(28.3,-14.,4.5));
#36611=CARTESIAN_POINT('',(9.4,-14.,6.));
#36612=CARTESIAN_POINT('',(20.,-14.,4.595));
#36613=CARTESIAN_POINT('Origin',(20.,-14.,5.2));
#36614=CARTESIAN_POINT('Origin',(20.,-14.,5.2));
#36615=CARTESIAN_POINT('Origin',(34.6,-13.,6.));
#36616=CARTESIAN_POINT('',(35.6,-13.,4.5));
#36617=CARTESIAN_POINT('',(35.6,-13.,6.));
#36618=CARTESIAN_POINT('Origin',(34.6,-13.,4.5));
#36619=CARTESIAN_POINT('Origin',(35.6,13.,6.));
#36620=CARTESIAN_POINT('',(35.6,13.,4.5));
#36621=CARTESIAN_POINT('',(35.6,13.,6.));
#36622=CARTESIAN_POINT('',(35.6,6.5,4.5));
#36623=CARTESIAN_POINT('Origin',(34.6,13.,6.));
#36624=CARTESIAN_POINT('',(34.6,14.,4.5));
#36625=CARTESIAN_POINT('',(34.6,14.,6.));
#36626=CARTESIAN_POINT('Origin',(34.6,13.,4.5));
#36627=CARTESIAN_POINT('Origin',(9.4,14.,6.));
#36628=CARTESIAN_POINT('',(20.,14.,4.595));
#36629=CARTESIAN_POINT('Origin',(20.,14.,5.2));
#36630=CARTESIAN_POINT('Origin',(20.,14.,5.2));
#36631=CARTESIAN_POINT('',(9.4,14.,4.5));
#36632=CARTESIAN_POINT('',(9.4,14.,6.));
#36633=CARTESIAN_POINT('',(15.7,14.,4.5));
#36634=CARTESIAN_POINT('Origin',(20.,14.59,5.2));
#36635=CARTESIAN_POINT('',(20.,15.2,4.595));
#36636=CARTESIAN_POINT('',(20.,14.59,4.595));
#36637=CARTESIAN_POINT('',(19.9223791265187,15.2,5.8));
#36638=CARTESIAN_POINT('Origin',(20.,15.2,5.2));
#36639=CARTESIAN_POINT('',(20.0776208734813,15.2,5.8));
#36640=CARTESIAN_POINT('Origin',(20.,15.4485281374238,5.2));
#36641=CARTESIAN_POINT('Origin',(20.,15.2,5.2));
#36642=CARTESIAN_POINT('Origin',(36.975,-7.025,0.));
#36643=CARTESIAN_POINT('',(37.,-7.05,2.05));
#36644=CARTESIAN_POINT('',(37.,-7.05,0.149999999999996));
#36645=CARTESIAN_POINT('',(37.,-7.05,0.));
#36646=CARTESIAN_POINT('',(36.975,-7.025,0.0896446609406665));
#36647=CARTESIAN_POINT('',(37.1479963503908,-7.19799635039082,0.507294796295184));
#36648=CARTESIAN_POINT('',(36.95,-7.,0.149999999999999));
#36649=CARTESIAN_POINT('',(35.3058538083499,-5.35585380834979,4.11932003440591));
#36650=CARTESIAN_POINT('',(36.95,-7.,2.));
#36651=CARTESIAN_POINT('',(36.95,-7.,0.));
#36652=CARTESIAN_POINT('',(36.95,-7.,2.));
#36653=CARTESIAN_POINT('Origin',(36.975,-6.6,2.025));
#36654=CARTESIAN_POINT('',(36.95,7.,2.));
#36655=CARTESIAN_POINT('',(36.95,-6.6,2.));
#36656=CARTESIAN_POINT('',(37.,7.05,2.05));
#36657=CARTESIAN_POINT('',(34.3666666666667,4.41666666666652,-0.583333333333435));
#36658=CARTESIAN_POINT('',(37.,-6.6,2.05));
#36659=CARTESIAN_POINT('Origin',(36.9823223304703,-9.9,0.107322330470332));
#36660=CARTESIAN_POINT('',(37.,-13.2,0.149999999999996));
#36661=CARTESIAN_POINT('',(37.,-9.9,0.149999999999996));
#36662=CARTESIAN_POINT('',(36.9646446609407,-13.2,0.0646446609406699));
#36663=CARTESIAN_POINT('',(37.,-13.2,0.149999999999996));
#36664=CARTESIAN_POINT('',(36.9646446609407,-7.03535533905933,0.0646446609406699));
#36665=CARTESIAN_POINT('',(36.9646446609407,-9.9,0.0646446609406684));
#36666=CARTESIAN_POINT('',(35.1179858427056,-8.88201415729434,-4.39358410311806));
#36667=CARTESIAN_POINT('Origin',(37.,-13.2,0.));
#36668=CARTESIAN_POINT('',(37.,7.05,0.150000000000001));
#36669=CARTESIAN_POINT('',(37.,7.05,0.));
#36670=CARTESIAN_POINT('',(37.,13.2,0.15));
#36671=CARTESIAN_POINT('',(37.,-9.9,0.149999999999996));
#36672=CARTESIAN_POINT('',(37.,13.2,5.80000000000001));
#36673=CARTESIAN_POINT('',(37.,13.2,0.));
#36674=CARTESIAN_POINT('',(37.,-13.2,5.8));
#36675=CARTESIAN_POINT('',(37.,-9.9,5.80000000000001));
#36676=CARTESIAN_POINT('',(37.,-13.2,0.));
#36677=CARTESIAN_POINT('Origin',(10.675,-7.01767766952966,0.107322330470336));
#36678=CARTESIAN_POINT('',(7.03535533905933,-7.03535533905933,0.0646446609406731));
#36679=CARTESIAN_POINT('',(10.675,-7.03535533905933,0.064644660940672));
#36680=CARTESIAN_POINT('',(7.025,-7.025,0.0896446609406749));
#36681=CARTESIAN_POINT('',(6.1707415527494,-6.17074155274938,2.15200699006485));
#36682=CARTESIAN_POINT('',(7.05,-7.,0.149999999999999));
#36683=CARTESIAN_POINT('',(7.24749543798848,-6.80250456201151,0.626796164898609));
#36684=CARTESIAN_POINT('',(10.675,-7.,0.149999999999999));
#36685=CARTESIAN_POINT('Origin',(7.025,-7.025,0.));
#36686=CARTESIAN_POINT('',(7.,-7.05,0.15));
#36687=CARTESIAN_POINT('',(8.11662550049235,-5.93337449950761,-2.54577242738026));
#36688=CARTESIAN_POINT('',(7.,-7.05,2.05));
#36689=CARTESIAN_POINT('',(7.,-7.05,0.));
#36690=CARTESIAN_POINT('',(7.05,-7.,2.));
#36691=CARTESIAN_POINT('',(7.,-7.05,2.05));
#36692=CARTESIAN_POINT('',(7.05,-7.,0.));
#36693=CARTESIAN_POINT('Origin',(7.01767766952966,9.9,0.107322330470337));
#36694=CARTESIAN_POINT('',(7.03535533905933,-13.2,0.0646446609406725));
#36695=CARTESIAN_POINT('',(7.03535533905933,9.9,0.0646446609406732));
#36696=CARTESIAN_POINT('',(7.,-13.2,0.15));
#36697=CARTESIAN_POINT('',(7.,-13.2,0.15));
#36698=CARTESIAN_POINT('',(7.,9.9,0.15));
#36699=CARTESIAN_POINT('Origin',(14.45,-7.05,0.05));
#36700=CARTESIAN_POINT('',(36.9353553390593,-7.06464466094067,0.0353553390593268));
#36701=CARTESIAN_POINT('',(36.9,-7.1,0.));
#36702=CARTESIAN_POINT('',(7.06464466094067,-7.06464466094067,0.0353553390593268));
#36703=CARTESIAN_POINT('',(18.225,-7.06464466094067,0.035355339059327));
#36704=CARTESIAN_POINT('',(7.,-7.,0.1));
#36705=CARTESIAN_POINT('Origin',(18.225,-7.10732233047034,0.0176776695296635));
#36706=CARTESIAN_POINT('',(7.1,-7.15,0.));
#36707=CARTESIAN_POINT('',(5.67626910198315,-3.71280955683808,1.42373089801684));
#36708=CARTESIAN_POINT('',(36.9,-7.15,0.));
#36709=CARTESIAN_POINT('',(35.8061358310127,-9.79082171216312,-1.09386416898729));
#36710=CARTESIAN_POINT('',(18.225,-7.15,0.));
#36711=CARTESIAN_POINT('Origin',(7.05,6.6,0.05));
#36712=CARTESIAN_POINT('',(7.1,-13.2,0.));
#36713=CARTESIAN_POINT('',(7.1,6.6,0.));
#36714=CARTESIAN_POINT('',(7.1,-13.2,0.));
#36715=CARTESIAN_POINT('Origin',(35.,13.2,5.98232233047034));
#36716=CARTESIAN_POINT('',(36.8853553390593,13.2,5.96464466094067));
#36717=CARTESIAN_POINT('',(36.8,13.2,6.));
#36718=CARTESIAN_POINT('',(35.,15.0853553390593,5.96464466094067));
#36719=CARTESIAN_POINT('Origin',(35.,13.2,5.96464466094067));
#36720=CARTESIAN_POINT('',(35.,15.0853553390593,5.96464466094067));
#36721=CARTESIAN_POINT('Origin',(36.8426776695297,-3.3,5.98232233047034));
#36722=CARTESIAN_POINT('',(36.8853553390593,-13.2,5.96464466094068));
#36723=CARTESIAN_POINT('',(36.8,-13.2,6.));
#36724=CARTESIAN_POINT('',(36.8853553390593,-3.3,5.96464466094067));
#36725=CARTESIAN_POINT('Origin',(35.,-13.2,5.98232233047034));
#36726=CARTESIAN_POINT('',(35.,-15.0853553390593,5.96464466094067));
#36727=CARTESIAN_POINT('',(35.,-15.,6.));
#36728=CARTESIAN_POINT('Origin',(35.,-13.2,5.96464466094067));
#36729=CARTESIAN_POINT('Origin',(18.75,-15.0426776695297,5.98232233047034));
#36730=CARTESIAN_POINT('',(9.,-15.0853553390593,5.96464466094067));
#36731=CARTESIAN_POINT('',(9.,-15.,6.));
#36732=CARTESIAN_POINT('',(18.75,-15.0853553390593,5.96464466094067));
#36733=CARTESIAN_POINT('Origin',(9.,-13.2,5.98232233047034));
#36734=CARTESIAN_POINT('',(7.11464466094067,-13.2,5.96464466094067));
#36735=CARTESIAN_POINT('',(7.2,-13.2,6.));
#36736=CARTESIAN_POINT('Origin',(9.,-13.2,5.96464466094067));
#36737=CARTESIAN_POINT('Origin',(7.15732233047034,3.3,5.98232233047034));
#36738=CARTESIAN_POINT('',(7.11464466094067,13.2,5.96464466094067));
#36739=CARTESIAN_POINT('',(7.2,13.2,6.));
#36740=CARTESIAN_POINT('',(7.11464466094067,3.3,5.96464466094067));
#36741=CARTESIAN_POINT('Origin',(9.,13.2,5.98232233047034));
#36742=CARTESIAN_POINT('',(9.,15.0853553390593,5.96464466094067));
#36743=CARTESIAN_POINT('',(9.,15.,6.));
#36744=CARTESIAN_POINT('Origin',(9.,13.2,5.96464466094067));
#36745=CARTESIAN_POINT('Origin',(25.25,15.0426776695297,5.98232233047034));
#36746=CARTESIAN_POINT('',(25.25,15.0853553390593,5.96464466094067));
#36747=CARTESIAN_POINT('Origin',(7.075,6.6,5.925));
#36748=CARTESIAN_POINT('',(7.03535533905933,13.2,5.88535533905933));
#36749=CARTESIAN_POINT('',(7.15,13.2,6.));
#36750=CARTESIAN_POINT('',(7.03535533905933,-13.2,5.88535533905933));
#36751=CARTESIAN_POINT('',(7.03535533905933,9.9,5.88535533905933));
#36752=CARTESIAN_POINT('',(7.,-13.2,5.85));
#36753=CARTESIAN_POINT('Origin',(9.,13.2,5.925));
#36754=CARTESIAN_POINT('',(9.,15.1646446609407,5.88535533905933));
#36755=CARTESIAN_POINT('',(9.,15.2,5.85));
#36756=CARTESIAN_POINT('Origin',(9.,13.2,5.88535533905933));
#36757=CARTESIAN_POINT('Origin',(28.5,15.125,5.925));
#36758=CARTESIAN_POINT('',(35.,15.1646446609407,5.88535533905933));
#36759=CARTESIAN_POINT('',(35.,15.2,5.85));
#36760=CARTESIAN_POINT('',(31.75,15.1646446609407,5.88535533905933));
#36761=CARTESIAN_POINT('Origin',(35.,13.2,5.925));
#36762=CARTESIAN_POINT('',(36.9646446609407,13.2,5.88535533905933));
#36763=CARTESIAN_POINT('',(37.,13.2,5.85));
#36764=CARTESIAN_POINT('Origin',(35.,13.2,5.88535533905933));
#36765=CARTESIAN_POINT('Origin',(7.01767766952966,9.9,5.84267766952966));
#36766=CARTESIAN_POINT('',(7.,-13.2,5.8));
#36767=CARTESIAN_POINT('',(7.,-13.2,5.8));
#36768=CARTESIAN_POINT('',(7.,13.2,5.8));
#36769=CARTESIAN_POINT('',(7.03535533905933,13.2,5.88535533905933));
#36770=CARTESIAN_POINT('',(7.,9.9,5.8));
#36771=CARTESIAN_POINT('Origin',(9.,-13.2,5.84267766952966));
#36772=CARTESIAN_POINT('',(9.,-15.2,5.8));
#36773=CARTESIAN_POINT('',(9.,-15.1646446609407,5.88535533905933));
#36774=CARTESIAN_POINT('',(9.,-15.2,5.8));
#36775=CARTESIAN_POINT('Origin',(9.,-13.2,5.88535533905933));
#36776=CARTESIAN_POINT('Origin',(9.,-13.2,5.8));
#36777=CARTESIAN_POINT('Origin',(12.25,-15.1823223304703,5.84267766952966));
#36778=CARTESIAN_POINT('',(19.9223791265187,-15.2,5.8));
#36779=CARTESIAN_POINT('',(20.0776208734813,-15.2,5.8));
#36780=CARTESIAN_POINT('Origin',(20.,-15.4485281374238,5.2));
#36781=CARTESIAN_POINT('',(35.,-15.2,5.8));
#36782=CARTESIAN_POINT('',(12.25,-15.2,5.8));
#36783=CARTESIAN_POINT('',(35.,-15.1646446609407,5.88535533905933));
#36784=CARTESIAN_POINT('',(35.,-15.2,5.8));
#36785=CARTESIAN_POINT('',(12.25,-15.1646446609407,5.88535533905933));
#36786=CARTESIAN_POINT('',(12.25,-15.2,5.8));
#36787=CARTESIAN_POINT('Origin',(35.,-13.2,5.84267766952966));
#36788=CARTESIAN_POINT('',(36.9646446609407,-13.2,5.88535533905933));
#36789=CARTESIAN_POINT('',(37.,-13.2,5.8));
#36790=CARTESIAN_POINT('Origin',(35.,-13.2,5.88535533905933));
#36791=CARTESIAN_POINT('Origin',(35.,-13.2,5.8));
#36792=CARTESIAN_POINT('Origin',(36.9823223304703,-9.9,5.84267766952967));
#36793=CARTESIAN_POINT('',(37.,13.2,5.80000000000001));
#36794=CARTESIAN_POINT('',(36.9646446609407,-9.9,5.88535533905933));
#36795=CARTESIAN_POINT('Origin',(35.,13.2,5.84267766952967));
#36796=CARTESIAN_POINT('',(35.,15.2,5.8));
#36797=CARTESIAN_POINT('',(35.,15.2,5.8));
#36798=CARTESIAN_POINT('Origin',(35.,13.2,5.8));
#36799=CARTESIAN_POINT('Origin',(31.75,15.1823223304703,5.84267766952966));
#36800=CARTESIAN_POINT('',(9.,15.2,5.8));
#36801=CARTESIAN_POINT('',(31.75,15.2,5.8));
#36802=CARTESIAN_POINT('',(9.,15.2,5.8));
#36803=CARTESIAN_POINT('',(31.75,15.2,5.8));
#36804=CARTESIAN_POINT('Origin',(9.,13.2,5.84267766952966));
#36805=CARTESIAN_POINT('Origin',(9.,13.2,5.8));
#36806=CARTESIAN_POINT('Origin',(9.,-15.2,0.));
#36807=CARTESIAN_POINT('',(9.,-15.2,0.150000000000001));
#36808=CARTESIAN_POINT('',(9.,-15.2,0.));
#36809=CARTESIAN_POINT('',(35.,-15.2,0.15));
#36810=CARTESIAN_POINT('',(12.25,-15.2,0.150000000000001));
#36811=CARTESIAN_POINT('',(35.,-15.2,0.));
#36812=CARTESIAN_POINT('',(20.,-15.2,4.595));
#36813=CARTESIAN_POINT('Origin',(20.,-15.2,5.2));
#36814=CARTESIAN_POINT('Origin',(20.,-15.2,5.2));
#36815=CARTESIAN_POINT('Origin',(9.,-13.2,0.));
#36816=CARTESIAN_POINT('',(7.,-13.2,0.));
#36817=CARTESIAN_POINT('Origin',(9.,-13.2,0.15));
#36818=CARTESIAN_POINT('Origin',(7.,13.2,0.));
#36819=CARTESIAN_POINT('',(7.,13.2,0.15));
#36820=CARTESIAN_POINT('',(7.,13.2,0.));
#36821=CARTESIAN_POINT('',(7.,7.05,0.15));
#36822=CARTESIAN_POINT('',(7.,9.9,0.15));
#36823=CARTESIAN_POINT('',(7.,7.05,2.05));
#36824=CARTESIAN_POINT('',(7.,7.05,0.));
#36825=CARTESIAN_POINT('',(7.,6.6,2.05));
#36826=CARTESIAN_POINT('Origin',(9.,13.2,0.));
#36827=CARTESIAN_POINT('',(9.,15.2,0.15));
#36828=CARTESIAN_POINT('',(9.,15.2,0.));
#36829=CARTESIAN_POINT('Origin',(9.,13.2,0.15));
#36830=CARTESIAN_POINT('Origin',(35.,15.2,0.));
#36831=CARTESIAN_POINT('',(35.,15.2,0.150000000000001));
#36832=CARTESIAN_POINT('',(35.,15.2,0.));
#36833=CARTESIAN_POINT('',(31.75,15.2,0.150000000000001));
#36834=CARTESIAN_POINT('Origin',(35.,-13.2,0.107322330470338));
#36835=CARTESIAN_POINT('',(35.,-15.1646446609407,0.0646446609406744));
#36836=CARTESIAN_POINT('',(35.,-15.2,0.15));
#36837=CARTESIAN_POINT('Origin',(35.,-13.2,0.0646446609406753));
#36838=CARTESIAN_POINT('Origin',(35.,-13.2,0.15));
#36839=CARTESIAN_POINT('Origin',(12.25,-15.1823223304703,0.107322330470337));
#36840=CARTESIAN_POINT('',(9.,-15.1646446609407,0.0646446609406738));
#36841=CARTESIAN_POINT('',(9.,-15.2,0.150000000000001));
#36842=CARTESIAN_POINT('',(12.25,-15.1646446609407,0.0646446609406733));
#36843=CARTESIAN_POINT('Origin',(9.,-13.2,0.107322330470337));
#36844=CARTESIAN_POINT('Origin',(9.,-13.2,0.0646446609406728));
#36845=CARTESIAN_POINT('Origin',(36.95,-6.6,0.05));
#36846=CARTESIAN_POINT('',(36.9,-13.2,0.));
#36847=CARTESIAN_POINT('',(36.9,-13.2,0.));
#36848=CARTESIAN_POINT('',(36.9,-6.6,0.));
#36849=CARTESIAN_POINT('Origin',(35.,-13.2,0.05));
#36850=CARTESIAN_POINT('',(35.,-15.1,0.));
#36851=CARTESIAN_POINT('',(35.,-15.1,0.));
#36852=CARTESIAN_POINT('Origin',(35.,-13.2,0.));
#36853=CARTESIAN_POINT('Origin',(15.5,-15.15,0.05));
#36854=CARTESIAN_POINT('',(9.,-15.1,0.));
#36855=CARTESIAN_POINT('',(9.,-15.1,0.));
#36856=CARTESIAN_POINT('',(15.5,-15.1,0.));
#36857=CARTESIAN_POINT('Origin',(9.,-13.2,0.05));
#36858=CARTESIAN_POINT('Origin',(9.,-13.2,0.));
#36859=CARTESIAN_POINT('Origin',(36.9353553390593,7.12588190451026,0.0353553390593253));
#36860=CARTESIAN_POINT('',(36.85,7.15,0.));
#36861=CARTESIAN_POINT('',(36.8741180954897,7.06464466094067,0.035355339059327));
#36862=CARTESIAN_POINT('',(36.85,7.15,0.));
#36863=CARTESIAN_POINT('',(36.9353553390593,7.12588190451026,0.0353553390593251));
#36864=CARTESIAN_POINT('',(36.9353553390593,7.12588190451026,0.0353553390593253));
#36865=CARTESIAN_POINT('',(36.8741180954897,7.06464466094067,0.0353553390593253));
#36866=CARTESIAN_POINT('Origin',(7.15,7.15,0.));
#36867=CARTESIAN_POINT('',(7.06464466094067,7.12588190451025,0.0353553390593283));
#36868=CARTESIAN_POINT('',(7.12588190451025,7.06464466094067,0.0353553390593273));
#36869=CARTESIAN_POINT('',(7.06464466094067,7.12588190451025,0.0353553390593291));
#36870=CARTESIAN_POINT('',(7.15,7.15,0.));
#36871=CARTESIAN_POINT('',(7.15,7.15,0.));
#36872=CARTESIAN_POINT('',(7.12588190451025,7.06464466094067,0.035355339059327));
#36873=CARTESIAN_POINT('Origin',(36.8926776695297,-3.3,0.0176776695296627));
#36874=CARTESIAN_POINT('',(36.85,13.2,0.));
#36875=CARTESIAN_POINT('',(36.9353553390593,13.2,0.035355339059327));
#36876=CARTESIAN_POINT('',(36.85,13.2,0.));
#36877=CARTESIAN_POINT('',(36.9353553390593,-3.3,0.0353553390593253));
#36878=CARTESIAN_POINT('',(36.85,-3.3,0.));
#36879=CARTESIAN_POINT('Origin',(35.,13.2,0.0176776695296633));
#36880=CARTESIAN_POINT('',(35.,15.05,0.));
#36881=CARTESIAN_POINT('',(35.,15.1353553390593,0.0353553390593202));
#36882=CARTESIAN_POINT('',(35.,15.05,0.));
#36883=CARTESIAN_POINT('Origin',(35.,13.2,0.0353553390593266));
#36884=CARTESIAN_POINT('Origin',(35.,13.2,0.));
#36885=CARTESIAN_POINT('Origin',(25.25,15.0926776695297,0.0176776695296636));
#36886=CARTESIAN_POINT('',(9.,15.05,0.));
#36887=CARTESIAN_POINT('',(9.,15.1353553390593,0.0353553390593265));
#36888=CARTESIAN_POINT('',(9.,15.05,0.));
#36889=CARTESIAN_POINT('',(25.25,15.1353553390593,0.0353553390593273));
#36890=CARTESIAN_POINT('',(25.25,15.05,0.));
#36891=CARTESIAN_POINT('Origin',(9.,13.2,0.017677669529664));
#36892=CARTESIAN_POINT('',(7.15,13.2,0.));
#36893=CARTESIAN_POINT('',(7.06464466094067,13.2,0.0353553390593274));
#36894=CARTESIAN_POINT('',(7.15,13.2,0.));
#36895=CARTESIAN_POINT('Origin',(9.,13.2,0.0353553390593279));
#36896=CARTESIAN_POINT('Origin',(9.,13.2,0.));
#36897=CARTESIAN_POINT('Origin',(7.10732233047034,3.3,0.0176776695296642));
#36898=CARTESIAN_POINT('',(7.15,3.3,0.));
#36899=CARTESIAN_POINT('',(7.06464466094067,3.3,0.0353553390593283));
#36900=CARTESIAN_POINT('Origin',(25.775,7.10732233047034,0.0176776695296635));
#36901=CARTESIAN_POINT('',(25.775,7.06464466094067,0.035355339059327));
#36902=CARTESIAN_POINT('',(25.775,7.15,0.));
#36903=CARTESIAN_POINT('Origin',(36.9545130195779,7.04548698042206,0.107322330470334));
#36904=CARTESIAN_POINT('',(36.9646446609407,7.09659258262892,0.0646446609406684));
#36905=CARTESIAN_POINT('',(36.9034074173711,7.03535533905933,0.064644660940667));
#36906=CARTESIAN_POINT('',(36.9646446609407,7.09659258262892,0.0646446609406675));
#36907=CARTESIAN_POINT('',(37.,7.05,0.149999999999996));
#36908=CARTESIAN_POINT('',(36.95,7.,0.149999999999999));
#36909=CARTESIAN_POINT('',(36.95,7.,0.149999999999999));
#36910=CARTESIAN_POINT('',(36.9034074173711,7.03535533905933,0.064644660940672));
#36911=CARTESIAN_POINT('Origin',(7.04548698042206,7.04548698042206,0.107322330470336));
#36912=CARTESIAN_POINT('',(7.05,7.,0.149999999999999));
#36913=CARTESIAN_POINT('',(7.0965925826289,7.03535533905933,0.064644660940672));
#36914=CARTESIAN_POINT('',(7.05,7.,0.149999999999999));
#36915=CARTESIAN_POINT('',(7.,7.05,0.15));
#36916=CARTESIAN_POINT('',(7.03535533905933,7.09659258262891,0.0646446609406737));
#36917=CARTESIAN_POINT('',(7.03535533905933,7.09659258262891,0.0646446609406732));
#36918=CARTESIAN_POINT('',(7.09659258262891,7.03535533905933,0.0646446609406715));
#36919=CARTESIAN_POINT('Origin',(7.025,7.025,0.));
#36920=CARTESIAN_POINT('',(7.05,7.,2.));
#36921=CARTESIAN_POINT('',(7.05,7.,0.));
#36922=CARTESIAN_POINT('',(7.05,7.,2.));
#36923=CARTESIAN_POINT('Origin',(7.025,6.6,2.025));
#36924=CARTESIAN_POINT('',(7.05,6.6,2.));
#36925=CARTESIAN_POINT('Origin',(7.01767766952966,9.9,0.107322330470337));
#36926=CARTESIAN_POINT('',(7.03535533905933,13.2,0.0646446609406729));
#36927=CARTESIAN_POINT('',(7.,13.2,0.15));
#36928=CARTESIAN_POINT('',(7.03535533905933,9.9,0.0646446609406732));
#36929=CARTESIAN_POINT('Origin',(9.,13.2,0.107322330470336));
#36930=CARTESIAN_POINT('',(9.,15.1646446609407,0.0646446609406726));
#36931=CARTESIAN_POINT('',(9.,15.2,0.15));
#36932=CARTESIAN_POINT('Origin',(9.,13.2,0.0646446609406726));
#36933=CARTESIAN_POINT('Origin',(31.75,15.1823223304703,0.107322330470337));
#36934=CARTESIAN_POINT('',(35.,15.1646446609407,0.0646446609406739));
#36935=CARTESIAN_POINT('',(35.,15.2,0.150000000000001));
#36936=CARTESIAN_POINT('',(31.75,15.1646446609407,0.0646446609406733));
#36937=CARTESIAN_POINT('Origin',(35.,13.2,0.107322330470338));
#36938=CARTESIAN_POINT('',(36.9646446609407,13.2,0.0646446609406714));
#36939=CARTESIAN_POINT('',(37.,13.2,0.15));
#36940=CARTESIAN_POINT('Origin',(35.,13.2,0.0646446609406769));
#36941=CARTESIAN_POINT('Origin',(35.,13.2,0.15));
#36942=CARTESIAN_POINT('Origin',(36.9823223304703,-9.9,0.107322330470332));
#36943=CARTESIAN_POINT('',(36.9646446609407,-9.9,0.0646446609406684));
#36944=CARTESIAN_POINT('Origin',(10.7352062072616,10.7352062072616,-3.60458758547682));
#36945=CARTESIAN_POINT('',(10.7658248290464,10.7045875854768,-3.60458758547682));
#36946=CARTESIAN_POINT('',(10.7045875854768,10.7658248290464,-3.60458758547682));
#36947=CARTESIAN_POINT('Origin',(33.325,7.01767766952966,0.107322330470336));
#36948=CARTESIAN_POINT('',(33.325,7.03535533905933,0.064644660940672));
#36949=CARTESIAN_POINT('',(33.325,7.,0.149999999999999));
#36950=CARTESIAN_POINT('Origin',(36.975,7.025,0.));
#36951=CARTESIAN_POINT('',(36.95,7.,0.));
#36952=CARTESIAN_POINT('Origin',(37.9814604594051,6.01853954059497,1.11207908118983));
#36953=CARTESIAN_POINT('',(38.0120790811898,6.04915816237976,1.11207908118983));
#36954=CARTESIAN_POINT('',(37.9508418376203,5.98792091881018,1.11207908118983));
#36955=CARTESIAN_POINT('Origin',(35.,13.2,0.05));
#36956=CARTESIAN_POINT('',(35.,15.1,0.));
#36957=CARTESIAN_POINT('',(36.9,13.2,0.));
#36958=CARTESIAN_POINT('Origin',(7.05,6.6,0.05));
#36959=CARTESIAN_POINT('',(7.1,13.2,0.));
#36960=CARTESIAN_POINT('Origin',(28.5,15.15,0.05));
#36961=CARTESIAN_POINT('',(9.,15.1,0.));
#36962=CARTESIAN_POINT('Origin',(9.,13.2,0.05));
#36963=CARTESIAN_POINT('Origin',(6.9,-7.,0.));
#36964=CARTESIAN_POINT('',(6.9,-7.,2.));
#36965=CARTESIAN_POINT('Origin',(22.,0.,2.));
#36966=CARTESIAN_POINT('',(37.1,7.,2.));
#36967=CARTESIAN_POINT('',(32.725,-1.07156594925393E-16,2.));
#36968=CARTESIAN_POINT('Origin',(33.6,0.,2.));
#36969=CARTESIAN_POINT('Origin',(37.1,7.,0.));
#36970=CARTESIAN_POINT('Origin',(22.,0.,0.));
#36971=CARTESIAN_POINT('Origin',(29.55,7.05,0.05));
#36972=CARTESIAN_POINT('Origin',(36.95,-6.6,0.05));
#36973=CARTESIAN_POINT('Origin',(22.,0.,0.));
#36974=CARTESIAN_POINT('Origin',(9.4,13.,4.5));
#36975=CARTESIAN_POINT('',(8.4,13.,4.5));
#36976=CARTESIAN_POINT('Origin',(8.7,13.,4.5));
#36977=CARTESIAN_POINT('Origin',(9.4,13.7,4.5));
#36978=CARTESIAN_POINT('Origin',(9.4,13.,4.5));
#36979=CARTESIAN_POINT('Origin',(15.7,13.7,4.5));
#36980=CARTESIAN_POINT('Origin',(34.6,13.7,4.5));
#36981=CARTESIAN_POINT('Origin',(34.6,13.,4.5));
#36982=CARTESIAN_POINT('Origin',(35.3,13.,4.5));
#36983=CARTESIAN_POINT('Origin',(35.3,6.5,4.5));
#36984=CARTESIAN_POINT('Origin',(35.3,-13.,4.5));
#36985=CARTESIAN_POINT('Origin',(34.6,-13.,4.5));
#36986=CARTESIAN_POINT('Origin',(34.6,-13.7,4.5));
#36987=CARTESIAN_POINT('Origin',(28.3,-13.7,4.5));
#36988=CARTESIAN_POINT('Origin',(9.4,-13.7,4.5));
#36989=CARTESIAN_POINT('Origin',(9.4,-13.,4.5));
#36990=CARTESIAN_POINT('',(8.4,-13.,4.5));
#36991=CARTESIAN_POINT('Origin',(8.7,-13.,4.5));
#36992=CARTESIAN_POINT('Origin',(9.4,-13.,4.5));
#36993=CARTESIAN_POINT('Origin',(8.7,-6.5,4.5));
#36994=CARTESIAN_POINT('',(8.4,-6.5,4.5));
#36995=CARTESIAN_POINT('Origin',(9.4,-13.,6.));
#36996=CARTESIAN_POINT('',(8.4,-13.,6.));
#36997=CARTESIAN_POINT('Origin',(8.4,-13.,6.));
#36998=CARTESIAN_POINT('',(8.4,13.,6.));
#36999=CARTESIAN_POINT('Origin',(9.4,13.,6.));
#37000=CARTESIAN_POINT('Origin',(9.4,-13.,5.925));
#37001=CARTESIAN_POINT('',(8.4,-13.,5.85));
#37002=CARTESIAN_POINT('Origin',(8.325,-6.5,5.925));
#37003=CARTESIAN_POINT('',(8.4,13.,5.85));
#37004=CARTESIAN_POINT('Origin',(9.4,13.,5.925));
#37005=CARTESIAN_POINT('',(9.4,14.,5.85));
#37006=CARTESIAN_POINT('Origin',(15.7,14.075,5.925));
#37007=CARTESIAN_POINT('Origin',(9.,-13.2,5.925));
#37008=CARTESIAN_POINT('',(9.,-15.2,5.85));
#37009=CARTESIAN_POINT('Origin',(15.5,-15.125,5.925));
#37010=CARTESIAN_POINT('',(35.,-15.2,5.85));
#37011=CARTESIAN_POINT('Origin',(35.,-13.2,5.925));
#37012=CARTESIAN_POINT('',(37.,-13.2,5.85));
#37013=CARTESIAN_POINT('Origin',(36.925,-6.6,5.925));
#37014=CARTESIAN_POINT('Origin',(35.,-13.2,0.));
#37015=CARTESIAN_POINT('Origin',(20.,-14.59,5.2));
#37016=CARTESIAN_POINT('',(20.,-14.59,4.595));
#37017=CARTESIAN_POINT('Origin',(33.6,0.,3.09));
#37018=CARTESIAN_POINT('',(32.725,-1.07156594925393E-16,3.09));
#37019=CARTESIAN_POINT('Origin',(29.,-9.2,2.04828269369554));
#37020=CARTESIAN_POINT('',(29.,-9.2,1.89656538739108));
#37021=CARTESIAN_POINT('',(28.7475,-9.2,2.04828269369554));
#37022=CARTESIAN_POINT('Origin',(29.,9.2,2.04828269369554));
#37023=CARTESIAN_POINT('',(29.,9.2,1.89656538739108));
#37024=CARTESIAN_POINT('',(28.7475,9.2,2.04828269369554));
#37025=CARTESIAN_POINT('Origin',(11.,-9.2,2.04828269369554));
#37026=CARTESIAN_POINT('',(11.,-9.2,1.89656538739108));
#37027=CARTESIAN_POINT('',(10.7475,-9.2,2.04828269369554));
#37028=CARTESIAN_POINT('Origin',(11.,9.2,2.04828269369554));
#37029=CARTESIAN_POINT('',(11.,9.2,1.89656538739108));
#37030=CARTESIAN_POINT('',(10.7475,9.2,2.04828269369554));
#37031=CARTESIAN_POINT('Origin',(21.,12.5,4.2));
#37032=CARTESIAN_POINT('',(21.,12.5,3.6));
#37033=CARTESIAN_POINT('',(21.,12.5,4.2));
#37034=CARTESIAN_POINT('',(21.,-12.5,3.6));
#37035=CARTESIAN_POINT('Origin',(19.,12.5,4.2));
#37036=CARTESIAN_POINT('',(21.,12.5,3.6));
#37037=CARTESIAN_POINT('Origin',(20.,0.,3.6));
#37038=CARTESIAN_POINT('Origin',(35.,13.2,0.));
#76618=UNCERTAINTY_MEASURE_WITH_UNIT(LENGTH_MEASURE(0.001),#76661,
'DISTANCE_ACCURACY_VALUE',
'Maximum model space distance between geometric entities at asserted c
onnectivities');
#76638=UNCERTAINTY_MEASURE_WITH_UNIT(LENGTH_MEASURE(0.001),#76661,
'DISTANCE_ACCURACY_VALUE',
'Maximum model space distance between geometric entities at asserted c
onnectivities');
#76640=(
GEOMETRIC_REPRESENTATION_CONTEXT(3)
GLOBAL_UNCERTAINTY_ASSIGNED_CONTEXT((#76618))
GLOBAL_UNIT_ASSIGNED_CONTEXT((#76661,#76663,#76664))
REPRESENTATION_CONTEXT('','3D')
);
#76660=(
GEOMETRIC_REPRESENTATION_CONTEXT(3)
GLOBAL_UNCERTAINTY_ASSIGNED_CONTEXT((#76638))
GLOBAL_UNIT_ASSIGNED_CONTEXT((#76661,#76663,#76664))
REPRESENTATION_CONTEXT('','3D')
);
#76661=(
LENGTH_UNIT()
NAMED_UNIT(*)
SI_UNIT(.CENTI.,.METRE.)
);
#76663=(
NAMED_UNIT(*)
PLANE_ANGLE_UNIT()
SI_UNIT($,.RADIAN.)
);
#76664=(
NAMED_UNIT(*)
SI_UNIT($,.STERADIAN.)
SOLID_ANGLE_UNIT()
);
#76666=SHAPE_DEFINITION_REPRESENTATION(#76687,#76736);
#76687=PRODUCT_DEFINITION_SHAPE('',$,#76758);
#76736=SHAPE_REPRESENTATION('',(#26906),#76640);
#76756=PRODUCT_DEFINITION_CONTEXT('part definition',#76821,'design');
#76758=PRODUCT_DEFINITION('2026-10-26-11-12-28-115',
'01_Base_Bed_Clamp_Block_Cast_Iron',#76779,#76756);
#76779=PRODUCT_DEFINITION_FORMATION('',$,#76824);
#76821=APPLICATION_CONTEXT(
'Core Data for Automotive Mechanical Design Process');
#76822=PRODUCT_CONTEXT('part definition',#76821,'mechanical');
#76824=PRODUCT('2026-10-26-11-12-28-115',
'01_Base_Bed_Clamp_Block_Cast_Iron',$,(#76822));
#76879=COLOUR_RGB('Dark Blue',0.08,0.2,0.34);
#76880=FILL_AREA_STYLE_COLOUR('',#76879);
#76881=FILL_AREA_STYLE('',(#76880));
#76882=SURFACE_STYLE_FILL_AREA(#76881);
#76883=SURFACE_SIDE_STYLE('',(#76882));
#76884=SURFACE_STYLE_USAGE(.BOTH.,#76883);
#76885=PRESENTATION_STYLE_ASSIGNMENT((#76884));
ENDSEC;
END-ISO-10303-21;
